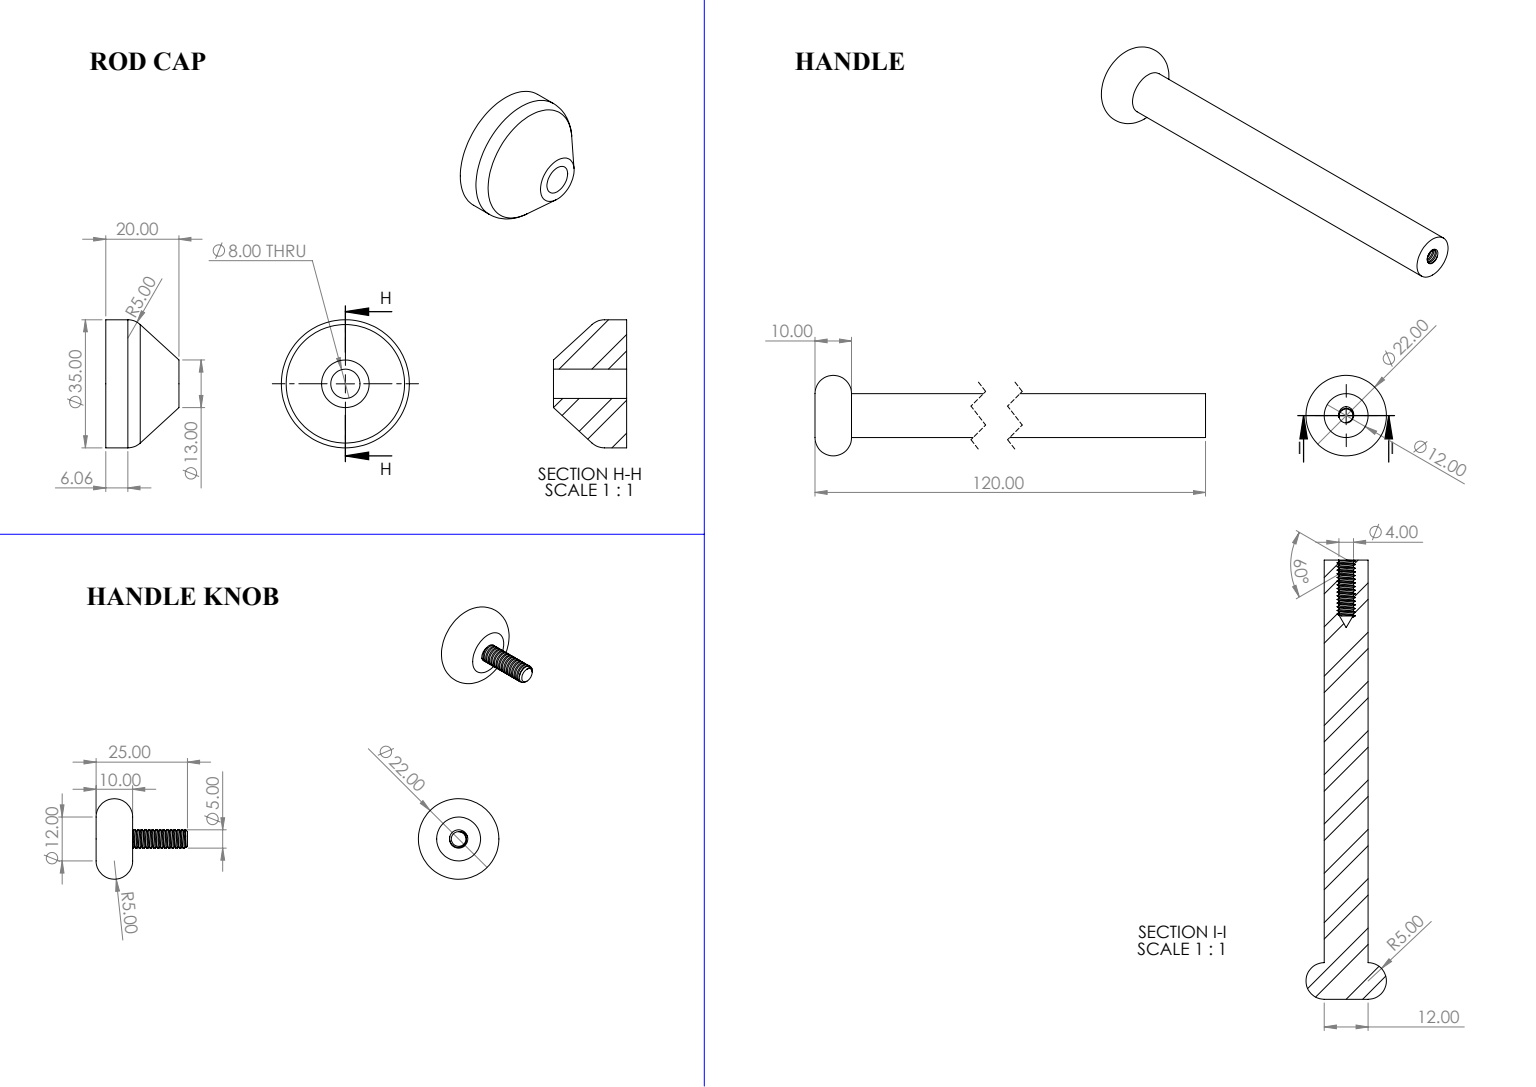
ISO-10303-21;
HEADER;
FILE_DESCRIPTION (('STEP AP214'),
    '1' );
FILE_NAME ('Handle knob.step',
    '2026-10-07T06:38:26',
    ( '' ),
    ( '' ),
    'SwSTEP 2.0',
    'SolidWorks 2021',
    '' );
FILE_SCHEMA (( 'AUTOMOTIVE_DESIGN' ));
ENDSEC;

DATA;
#8=CARTESIAN_POINT ( 'NONE',  ( 11.81249999999999822, -2.649519052838298805, 1.097466725451559322 ) ) ;
#12=CARTESIAN_POINT ( 'NONE',  ( 18.18750000000005684, 0.8284271247463557142, 1.999999999999971800 ) ) ;
#24=CARTESIAN_POINT ( 'NONE',  ( 15.64882486540532547, 2.500000000000084821, -1.035533905932929599 ) ) ;
#43=VECTOR ( 'NONE', #27184, 1000.000000000000000 ) ;
#80=SURFACE_SIDE_STYLE ('',( #6693 ) ) ;
#85=CARTESIAN_POINT ( 'NONE',  ( 19.25000000000009948, 1.110223024625156540E-13, 1.999999999999946265 ) ) ;
#100=CARTESIAN_POINT ( 'NONE',  ( 23.03867513459492855, 2.220446049250313081E-13, -2.500000000000057732 ) ) ;
#114=CARTESIAN_POINT ( 'NONE',  ( 9.937500000000083489, -1.097466725451379244, 2.649519052838238409 ) ) ;
#115=UNCERTAINTY_MEASURE_WITH_UNIT (LENGTH_MEASURE( 1.000000000000000082E-05 ), #12056, 'distance_accuracy_value', 'NONE');
#119=CARTESIAN_POINT ( 'NONE',  ( 23.66367513459491434, -1.767766952966209892, 1.767766952966376426 ) ) ;
#123=ORIENTED_EDGE ( 'NONE', *, *, #24115, .F. ) ;
#129=CARTESIAN_POINT ( 'NONE',  ( 21.62500000000011724, 1.110223024625156540E-13, 2.649519052838167354 ) ) ;
#153=CARTESIAN_POINT ( 'NONE',  ( 21.25000000000013145, -1.873492889144845464, -1.873492889145178530 ) ) ;
#161=CARTESIAN_POINT ( 'NONE',  ( 22.21132486540528106, -2.499999999999780176, -1.110223024625156540E-13 ) ) ;
#166=CARTESIAN_POINT ( 'NONE',  ( 20.85117513459493921, -2.499999999999844569, -1.035533905932809473 ) ) ;
#173=CARTESIAN_POINT ( 'NONE',  ( 19.75000000000009948, 1.665334536937734811E-13, -2.000000000000001776 ) ) ;
#178=CARTESIAN_POINT ( 'NONE',  ( 13.03867513459488947, 5.551115123125782702E-14, -2.500000000000002220 ) ) ;
#220=CARTESIAN_POINT ( 'NONE',  ( 16.37500000000008527, -1.414213562373090038, 1.414213562373034527 ) ) ;
#223=FACE_OUTER_BOUND ( 'NONE', #11618, .T. ) ;
#232=CARTESIAN_POINT ( 'NONE',  ( 22.87500000000000711, 1.414213562373312083, -1.414213562373090038 ) ) ;
#256=CARTESIAN_POINT ( 'NONE',  ( 13.83632486540523132, 1.767766952966376426, 1.767766952966376426 ) ) ;
#260=CARTESIAN_POINT ( 'NONE',  ( 23.37500000000000711, -1.414213562373090038, 1.414213562373034527 ) ) ;
#262=EDGE_CURVE ( 'NONE', #25850, #8065, #1532, .T. ) ;
#274=STYLED_ITEM ( 'NONE', ( #25687 ), #21644 ) ;
#276=CARTESIAN_POINT ( 'NONE',  ( 19.25000000000009948, 1.873492889145067508, -1.873492889144956486 ) ) ;
#295=CARTESIAN_POINT ( 'NONE',  ( 17.56250000000009592, 2.649519052838419153, -1.097466725451619718 ) ) ;
#305=VERTEX_POINT ( 'NONE', #20290 ) ;
#315=CARTESIAN_POINT ( 'NONE',  ( 10.25000000000000888, 1.873492889144956486, -1.873492889144900975 ) ) ;
#317=CARTESIAN_POINT ( 'NONE',  ( 19.31250000000010303, -0.8284271247459350507, 2.000000000000091926 ) ) ;
#335=PRESENTATION_STYLE_ASSIGNMENT (( #28879 ) ) ;
#377=CARTESIAN_POINT ( 'NONE',  ( 20.25000000000015632, 1.110223024625156540E-13, 1.999999999999946265 ) ) ;
#408=DIRECTION ( 'NONE',  ( -8.326672684688675286E-17, -2.081668171172168821E-17, 1.000000000000000000 ) ) ;
#416=CARTESIAN_POINT ( 'NONE',  ( 18.12500000000011369, 1.110223024625156540E-13, -2.649519052838278377 ) ) ;
#443=EDGE_LOOP ( 'NONE', ( #123, #12542, #25078, #1896 ) ) ;
#455=CARTESIAN_POINT ( 'NONE',  ( 10.93750000000009948, 2.000000000000091926, -0.8284271247462354770 ) ) ;
#456=ORIENTED_EDGE ( 'NONE', *, *, #9428, .T. ) ;
#458=CARTESIAN_POINT ( 'NONE',  ( 12.37500000000010836, 2.649519052838500421, 0.000000000000000000 ) ) ;
#462=CARTESIAN_POINT ( 'NONE',  ( 20.43750000000014566, -1.999999999999911626, 0.8284271247462354770 ) ) ;
#465=CARTESIAN_POINT ( 'NONE',  ( 22.97617513459487881, -1.035533905932689347, -2.500000000000024425 ) ) ;
#473=EDGE_CURVE ( 'NONE', #2749, #5395, #21945, .T. ) ;
#475=CARTESIAN_POINT ( 'NONE',  ( 15.71132486540535744, 2.500000000000113243, -1.110223024625156540E-13 ) ) ;
#482=CARTESIAN_POINT ( 'NONE',  ( 11.93750000000008527, 2.000000000000091926, -0.8284271247462354770 ) ) ;
#526=CARTESIAN_POINT ( 'NONE',  ( 22.00000000000010303, 2.000000000000168310, 0.000000000000000000 ) ) ;
#531=AXIS2_PLACEMENT_3D ( 'NONE', #29230, #26925, #12705 ) ;
#532=EDGE_CURVE ( 'NONE', #23217, #14931, #6701, .T. ) ;
#554=CARTESIAN_POINT ( 'NONE',  ( 23.50000000000010303, -1.999999999999779732, -5.551115123125782702E-14 ) ) ;
#566=VERTEX_POINT ( 'NONE', #11935 ) ;
#569=CARTESIAN_POINT ( 'NONE',  ( 16.87499999999997158, -2.649519052838222866, 0.000000000000000000 ) ) ;
#576=AXIS2_PLACEMENT_3D ( 'NONE', #8205, #17621, #15159 ) ;
#595=ORIENTED_EDGE ( 'NONE', *, *, #5857, .F. ) ;
#599=( BOUNDED_CURVE ( )  B_SPLINE_CURVE ( 2, ( #12471, #25953, #21667, #4903, #7659, #2902, #14759, #17068, #757 ),
 .UNSPECIFIED., .F., .T. ) 
 B_SPLINE_CURVE_WITH_KNOTS ( ( 3, 2, 2, 2, 3 ),
 ( 0.4531250000000000000, 0.4609375000000000000, 0.4687500000000000000, 0.4765625000000000000, 0.4843750000000000000 ),
 .UNSPECIFIED. ) 
 CURVE ( )  GEOMETRIC_REPRESENTATION_ITEM ( )  RATIONAL_B_SPLINE_CURVE ( ( 1.000000000000000000, 0.9238795325112867385, 1.000000000000000000, 0.9238795325112867385, 1.000000000000000000, 0.9238795325112867385, 1.000000000000000000, 0.9238795325112867385, 1.000000000000000000 ) ) 
 REPRESENTATION_ITEM ( '' )  );
#604=CARTESIAN_POINT ( 'NONE',  ( 22.58632486540529527, 1.767766952966487448, -1.767766952966431937 ) ) ;
#611=CARTESIAN_POINT ( 'NONE',  ( 11.12500000000010658, 1.414213562373201061, 1.414213562373034527 ) ) ;
#620=CARTESIAN_POINT ( 'NONE',  ( 20.75000000000012790, 1.665334536937734811E-13, -2.000000000000001776 ) ) ;
#623=CARTESIAN_POINT ( 'NONE',  ( 10.00000000000014744, 1.110223024625156540E-13, -5.551115123125782702E-14 ) ) ;
#625=CARTESIAN_POINT ( 'NONE',  ( -2.081668171172168020E-16, -5.204170427930420051E-17, 2.499999999999999112 ) ) ;
#626=CARTESIAN_POINT ( 'NONE',  ( 15.53867513459491967, 1.110223024625156540E-13, 2.499999999999835687 ) ) ;
#641=CARTESIAN_POINT ( 'NONE',  ( 12.06249999999996447, 2.000000000000091926, 0.8284271247461753029 ) ) ;
#644=CARTESIAN_POINT ( 'NONE',  ( 20.46132486540533435, 1.110223024625156540E-13, -2.500000000000057732 ) ) ;
#675=CARTESIAN_POINT ( 'NONE',  ( 17.31250000000004263, -0.8284271247461152399, 2.000000000000091926 ) ) ;
#687=CARTESIAN_POINT ( 'NONE',  ( 23.00000000000013145, 2.000000000000168310, 0.000000000000000000 ) ) ;
#699=( NAMED_UNIT ( * ) SI_UNIT ( $, .STERADIAN. ) SOLID_ANGLE_UNIT ( ) );
#710=CARTESIAN_POINT ( 'NONE',  ( 24.87500000000009237, 1.414213562373312083, -1.414213562373145550 ) ) ;
#725=CARTESIAN_POINT ( 'NONE',  ( 20.18750000000012079, 1.097466725451679892, -2.649519052838238409 ) ) ;
#736=ORIENTED_EDGE ( 'NONE', *, *, #27454, .T. ) ;
#751=CARTESIAN_POINT ( 'NONE',  ( 17.06250000000010303, -2.649519052838178457, 1.097466725451559322 ) ) ;
#757=CARTESIAN_POINT ( 'NONE',  ( 17.53867513459494987, 1.665334536937734811E-13, 2.499999999999946709 ) ) ;
#760=ORIENTED_EDGE ( 'NONE', *, *, #21946, .T. ) ;
#773=CARTESIAN_POINT ( 'NONE',  ( 17.00000000000015277, 2.000000000000112799, 0.000000000000000000 ) ) ;
#809=EDGE_CURVE ( 'NONE', #26790, #13355, #14385, .T. ) ;
#829=CARTESIAN_POINT ( 'NONE',  ( 17.06250000000001066, 2.000000000000151879, 0.8284271247461753029 ) ) ;
#833=CARTESIAN_POINT ( 'NONE',  ( 15.50000000000023626, 1.873492889145123019, 1.873492889144845464 ) ) ;
#835=EDGE_CURVE ( 'NONE', #29880, #28765, #16801, .T. ) ;
#861=CARTESIAN_POINT ( 'NONE',  ( 18.81250000000011013, -2.649519052838178457, 1.097466725451379244 ) ) ;
#881=DIRECTION ( 'NONE',  ( -1.000000000000000000, -1.665334536937731113E-16, 1.526556658859586792E-16 ) ) ;
#886=VERTEX_POINT ( 'NONE', #10157 ) ;
#887=CARTESIAN_POINT ( 'NONE',  ( 19.18750000000007461, -2.649519052838178457, -1.097466725451499370 ) ) ;
#920=CARTESIAN_POINT ( 'NONE',  ( 13.08632486540528461, -1.767766952966265404, 1.767766952966320915 ) ) ;
#930=CARTESIAN_POINT ( 'NONE',  ( 11.21132486540529705, -2.499999999999891198, -5.551115123125782702E-14 ) ) ;
#935=CARTESIAN_POINT ( 'NONE',  ( 25.25000000000015987, 1.873492889145067508, -1.873492889144956486 ) ) ;
#937=DIRECTION ( 'NONE',  ( -8.326672684688675286E-17, -2.081668171172168821E-17, 1.000000000000000000 ) ) ;
#971=CARTESIAN_POINT ( 'NONE',  ( 18.12500000000000355, 1.414213562373090038, 1.414213562373090038 ) ) ;
#981=DIRECTION ( 'NONE',  ( -8.326672684688675286E-17, -2.081668171172168821E-17, 1.000000000000000000 ) ) ;
#984=PLANE ( 'NONE',  #25487 ) ;
#996=CARTESIAN_POINT ( 'NONE',  ( 18.21132486540530238, -2.499999999999835687, -2.220446049250313081E-13 ) ) ;
#997=CARTESIAN_POINT ( 'NONE',  ( 10.77382486540524376, 2.499999999999964473, 1.035533905932689347 ) ) ;
#999=ORIENTED_EDGE ( 'NONE', *, *, #22038, .F. ) ;
#1028=DIRECTION ( 'NONE',  ( -1.000000000000000000, -1.665334536937731113E-16, 1.526556658859586792E-16 ) ) ;
#1035=( BOUNDED_CURVE ( )  B_SPLINE_CURVE ( 2, ( #20444, #22610, #6457, #17710, #18023, #8300, #10800, #6304, #22145 ),
 .UNSPECIFIED., .F., .T. ) 
 B_SPLINE_CURVE_WITH_KNOTS ( ( 3, 2, 2, 2, 3 ),
 ( 0.04687500000000000000, 0.05468750000000000000, 0.06250000000000000000, 0.07031250000000000000, 0.07812500000000000000 ),
 .UNSPECIFIED. ) 
 CURVE ( )  GEOMETRIC_REPRESENTATION_ITEM ( )  RATIONAL_B_SPLINE_CURVE ( ( 1.000000000000000000, 0.9238795325112867385, 1.000000000000000000, 0.9238795325112867385, 1.000000000000000000, 0.9238795325112867385, 1.000000000000000000, 0.9238795325112867385, 1.000000000000000000 ) ) 
 REPRESENTATION_ITEM ( '' )  );
#1038=CARTESIAN_POINT ( 'NONE',  ( 11.16367513459498539, 1.767766952966431937, -1.767766952966431937 ) ) ;
#1042=CARTESIAN_POINT ( 'NONE',  ( 13.50000000000006750, 1.873492889145123019, -1.873492889145011997 ) ) ;
#1084=CARTESIAN_POINT ( 'NONE',  ( 16.83632486540531659, 1.767766952966487448, 1.767766952966320915 ) ) ;
#1089=CARTESIAN_POINT ( 'NONE',  ( 10.43750000000004619, -1.999999999999851674, 0.8284271247461753029 ) ) ;
#1093=CARTESIAN_POINT ( 'NONE',  ( 20.96132486540536277, 5.551115123125782702E-14, 2.500000000000002220 ) ) ;
#1096=CARTESIAN_POINT ( 'NONE',  ( 10.06250000000005151, 2.000000000000212275, 0.8284271247461152399 ) ) ;
#1099=FACE_OUTER_BOUND ( 'NONE', #25635, .T. ) ;
#1113=CARTESIAN_POINT ( 'NONE',  ( 15.12500000000000000, 1.414213562373201061, 1.414213562373034527 ) ) ;
#1125=CARTESIAN_POINT ( 'NONE',  ( 15.31250000000006928, -0.8284271247461753029, 1.999999999999911626 ) ) ;
#1148=CARTESIAN_POINT ( 'NONE',  ( 10.89882486540524198, 1.035533905932749299, 2.499999999999904521 ) ) ;
#1155=ADVANCED_BREP_SHAPE_REPRESENTATION ( '', ( #4002, #18805 ), #12932 ) ;
#1156=( BOUNDED_CURVE ( )  B_SPLINE_CURVE ( 2, ( #15701, #3965, #25011, #22735, #10302, #12938, #19665, #29006, #22274 ),
 .UNSPECIFIED., .F., .F. ) 
 B_SPLINE_CURVE_WITH_KNOTS ( ( 3, 2, 2, 2, 3 ),
 ( 0.2656250000000000000, 0.2734375000000000000, 0.2812500000000000000, 0.2890625000000000000, 0.2968750000000000000 ),
 .UNSPECIFIED. ) 
 CURVE ( )  GEOMETRIC_REPRESENTATION_ITEM ( )  RATIONAL_B_SPLINE_CURVE ( ( 1.000000000000000000, 0.9238795325112867385, 1.000000000000000000, 0.9238795325112867385, 1.000000000000000000, 0.9238795325112867385, 1.000000000000000000, 0.9238795325112867385, 1.000000000000000000 ) ) 
 REPRESENTATION_ITEM ( '' )  );
#1171=CARTESIAN_POINT ( 'NONE',  ( 10.27382486540518869, -2.499999999999844569, -1.035533905932809473 ) ) ;
#1182=CARTESIAN_POINT ( 'NONE',  ( 14.68750000000004796, 2.649519052838478661, 1.097466725451439196 ) ) ;
#1194=VERTEX_POINT ( 'NONE', #13469 ) ;
#1202=CARTESIAN_POINT ( 'NONE',  ( 14.81250000000010658, 0.8284271247463557142, -2.000000000000031530 ) ) ;
#1221=CARTESIAN_POINT ( 'NONE',  ( 24.12500000000011724, -2.649519052838167354, 0.000000000000000000 ) ) ;
#1225=ADVANCED_FACE ( 'NONE', ( #2223 ), #14094, .T. ) ;
#1232=CARTESIAN_POINT ( 'NONE',  ( 19.53867513459495342, 5.551115123125782702E-14, 2.500000000000002220 ) ) ;
#1239=CARTESIAN_POINT ( 'NONE',  ( 24.62500000000000711, 1.110223024625156540E-13, 2.649519052838056332 ) ) ;
#1242=CARTESIAN_POINT ( 'NONE',  ( 2.081668171172167281E-16, 3.582034040661430693E-16, -2.499999999999999112 ) ) ;
#1267=CARTESIAN_POINT ( 'NONE',  ( 15.93749999999996980, 2.000000000000091926, -0.8284271247462955401 ) ) ;
#1275=B_SPLINE_CURVE_WITH_KNOTS ( 'NONE', 3,
 ( #25498, #22914, #30115, #6462, #15730, #4464, #25040, #13891, #15888, #15580, #24893, #11260, #11103, #29807, #23230, #3842, #22615, #20610 ),
 .UNSPECIFIED., .F., .F.,
 ( 4, 2, 2, 2, 2, 2, 2, 2, 4 ),
 ( 0.001391798398341157015, 0.001904360710870518173, 0.002416923023399879331, 0.002929485335929240489, 0.003442047648458601648, 0.003954609960987962372, 0.004467172273517323530, 0.004979734586046684688, 0.005492296898576045847 ),
 .UNSPECIFIED. ) ;
#1278=CARTESIAN_POINT ( 'NONE',  ( 18.18750000000005684, 0.8284271247463557142, 1.999999999999971800 ) ) ;
#1298=( BOUNDED_CURVE ( )  B_SPLINE_CURVE ( 2, ( #8723, #27280, #10584, #3789, #10750, #8562, #6254, #15672, #29438 ),
 .UNSPECIFIED., .F., .T. ) 
 B_SPLINE_CURVE_WITH_KNOTS ( ( 3, 2, 2, 2, 3 ),
 ( 0.2031250000000000000, 0.2109375000000000000, 0.2187500000000000000, 0.2265625000000000000, 0.2343750000000000000 ),
 .UNSPECIFIED. ) 
 CURVE ( )  GEOMETRIC_REPRESENTATION_ITEM ( )  RATIONAL_B_SPLINE_CURVE ( ( 1.000000000000000000, 0.9238795325112867385, 1.000000000000000000, 0.9238795325112867385, 1.000000000000000000, 0.9238795325112867385, 1.000000000000000000, 0.9238795325112867385, 1.000000000000000000 ) ) 
 REPRESENTATION_ITEM ( '' )  );
#1310=CARTESIAN_POINT ( 'NONE',  ( 0.000000000000000000, 0.000000000000000000, 0.000000000000000000 ) ) ;
#1314=UNCERTAINTY_MEASURE_WITH_UNIT (LENGTH_MEASURE( 1.000000000000000082E-05 ), #17406, 'distance_accuracy_value', 'NONE');
#1327=CARTESIAN_POINT ( 'NONE',  ( 22.66367513459499605, -1.767766952966265404, 1.767766952966376426 ) ) ;
#1338=CARTESIAN_POINT ( 'NONE',  ( 23.89882486540529882, 1.035533905932809473, 2.499999999999844569 ) ) ;
#1344=CARTESIAN_POINT ( 'NONE',  ( 14.50000000000012434, 1.873492889145067508, -1.873492889144956486 ) ) ;
#1370=CARTESIAN_POINT ( 'NONE',  ( 16.68750000000013856, -0.8284271247461753029, -2.000000000000151879 ) ) ;
#1385=CARTESIAN_POINT ( 'NONE',  ( 17.72617513459489658, -2.499999999999964473, 1.035533905932749299 ) ) ;
#1393=CARTESIAN_POINT ( 'NONE',  ( 19.72617513459489658, -2.499999999999964473, 1.035533905932809473 ) ) ;
#1417=CARTESIAN_POINT ( 'NONE',  ( 10.35117513459487704, 2.500000000000084821, 1.035533905932689347 ) ) ;
#1427=CARTESIAN_POINT ( 'NONE',  ( 14.68750000000004796, -0.8284271247460552878, -1.999999999999971800 ) ) ;
#1428=ORIENTED_EDGE ( 'NONE', *, *, #835, .F. ) ;
#1439=CARTESIAN_POINT ( 'NONE',  ( 15.81250000000000000, 0.8284271247462354770, -2.000000000000151879 ) ) ;
#1442=CARTESIAN_POINT ( 'NONE',  ( 14.68749999999998579, -1.097466725451499370, 2.649519052838298805 ) ) ;
#1469=ORIENTED_EDGE ( 'NONE', *, *, #28809, .T. ) ;
#1494=CARTESIAN_POINT ( 'NONE',  ( 15.81250000000009237, 1.097466725451619718, 2.649519052838419153 ) ) ;
#1507=AXIS2_PLACEMENT_3D ( 'NONE', #7070, #30110, #16484 ) ;
#1520=CARTESIAN_POINT ( 'NONE',  ( 13.25000000000017764, 5.551115123125782702E-14, 1.999999999999890754 ) ) ;
#1524=VECTOR ( 'NONE', #23636, 1000.000000000000000 ) ;
#1532=LINE ( 'NONE', #1995, #6368 ) ;
#1536=ORIENTED_EDGE ( 'NONE', *, *, #23552, .F. ) ;
#1537=CARTESIAN_POINT ( 'NONE',  ( 24.25000000000010658, -1.873492889144789952, -1.873492889145123019 ) ) ;
#1561=CARTESIAN_POINT ( 'NONE',  ( 24.43750000000014921, -1.999999999999851674, 0.8284271247462354770 ) ) ;
#1573=CARTESIAN_POINT ( 'NONE',  ( 14.22617513459491256, 2.500000000000144773, -1.035533905932689347 ) ) ;
#1574=VERTEX_POINT ( 'NONE', #20789 ) ;
#1578=( BOUNDED_CURVE ( )  B_SPLINE_CURVE ( 2, ( #24390, #7794, #1038, #19787, #25134, #13365, #5946, #20258, #27140 ),
 .UNSPECIFIED., .F., .T. ) 
 B_SPLINE_CURVE_WITH_KNOTS ( ( 3, 2, 2, 2, 3 ),
 ( 0.07812500000000000000, 0.08593750000000000000, 0.09375000000000000000, 0.1015625000000000000, 0.1093750000000000000 ),
 .UNSPECIFIED. ) 
 CURVE ( )  GEOMETRIC_REPRESENTATION_ITEM ( )  RATIONAL_B_SPLINE_CURVE ( ( 1.000000000000000000, 0.9238795325112867385, 1.000000000000000000, 0.9238795325112867385, 1.000000000000000000, 0.9238795325112867385, 1.000000000000000000, 0.9238795325112867385, 1.000000000000000000 ) ) 
 REPRESENTATION_ITEM ( '' )  );
#1583=AXIS2_PLACEMENT_3D ( 'NONE', #28607, #19132, #14405 ) ;
#1594=CARTESIAN_POINT ( 'NONE',  ( 13.75000000000006750, 2.220446049250313081E-13, -2.000000000000001776 ) ) ;
#1597=CARTESIAN_POINT ( 'NONE',  ( 14.43750000000004974, 2.649519052838419153, 1.097466725451439196 ) ) ;
#1606=CARTESIAN_POINT ( 'NONE',  ( 17.89882486540517093, 1.035533905932749299, 2.499999999999964473 ) ) ;
#1612=TOROIDAL_SURFACE ( 'NONE', #14425, 6.000000000000000888, 5.000000000000000888 ) ;
#1617=CARTESIAN_POINT ( 'NONE',  ( 20.81250000000014211, 0.8284271247461753029, -2.000000000000091926 ) ) ;
#1626=ORIENTED_EDGE ( 'NONE', *, *, #5088, .F. ) ;
#1628=CARTESIAN_POINT ( 'NONE',  ( 16.68750000000013856, -1.097466725451439196, 2.649519052838178457 ) ) ;
#1636=ORIENTED_EDGE ( 'NONE', *, *, #13213, .F. ) ;
#1654=CARTESIAN_POINT ( 'NONE',  ( 14.06250000000011546, -2.649519052838238409, 1.097466725451559322 ) ) ;
#1691=EDGE_CURVE ( 'NONE', #24822, #4865, #27940, .T. ) ;
#1702=CARTESIAN_POINT ( 'NONE',  ( 15.02382486540530238, -1.035533905932568999, 2.499999999999784173 ) ) ;
#1714=CARTESIAN_POINT ( 'NONE',  ( 22.31250000000002842, -0.8284271247460552878, 2.000000000000031530 ) ) ;
#1721=CARTESIAN_POINT ( 'NONE',  ( 12.03867513459491789, 1.665334536937734811E-13, -2.500000000000057732 ) ) ;
#1727=CYLINDRICAL_SURFACE ( 'NONE', #6676, 2.499999999999999112 ) ;
#1742=CARTESIAN_POINT ( 'NONE',  ( 11.93750000000008527, 2.000000000000091926, -0.8284271247462354770 ) ) ;
#1744=EDGE_CURVE ( 'NONE', #13355, #26790, #5902, .T. ) ;
#1746=CARTESIAN_POINT ( 'NONE',  ( 18.16367513459488237, 1.767766952966487448, -1.767766952966487448 ) ) ;
#1752=CARTESIAN_POINT ( 'NONE',  ( 0.000000000000000000, 0.000000000000000000, 0.000000000000000000 ) ) ;
#1767=CARTESIAN_POINT ( 'NONE',  ( 20.12500000000011369, 1.414213562373201061, 1.414213562373034527 ) ) ;
#1773=CARTESIAN_POINT ( 'NONE',  ( 14.77382486540530770, 2.500000000000144773, 1.035533905932689347 ) ) ;
#1778=EDGE_LOOP ( 'NONE', ( #21927, #2761, #24888, #28248 ) ) ;
#1793=CARTESIAN_POINT ( 'NONE',  ( 10.39882486540515849, -1.035533905932629173, -2.500000000000024425 ) ) ;
#1802=CARTESIAN_POINT ( 'NONE',  ( 11.62500000000010658, 2.649519052838444910, -1.110223024625156540E-13 ) ) ;
#1806=VERTEX_POINT ( 'NONE', #14612 ) ;
#1817=EDGE_CURVE ( 'NONE', #9159, #21560, #599, .T. ) ;
#1819=CARTESIAN_POINT ( 'NONE',  ( 10.37500000000005151, -1.414213562373034527, 1.414213562372756972 ) ) ;
#1828=CARTESIAN_POINT ( 'NONE',  ( 11.62499999999999645, -1.414213562373090038, -1.414213562373090038 ) ) ;
#1846=CARTESIAN_POINT ( 'NONE',  ( 21.12500000000011724, -2.649519052838222866, 0.000000000000000000 ) ) ;
#1866=CARTESIAN_POINT ( 'NONE',  ( 23.56250000000009948, -1.999999999999851674, -0.8284271247462354770 ) ) ;
#1879=DIRECTION ( 'NONE',  ( -1.000000000000000000, -1.665334536937731113E-16, 1.526556658859586792E-16 ) ) ;
#1893=SHAPE_REPRESENTATION ( 'Handle knob', ( #18805 ), #12932 ) ;
#1896=ORIENTED_EDGE ( 'NONE', *, *, #30228, .T. ) ;
#1897=CARTESIAN_POINT ( 'NONE',  ( 13.37500000000019185, -1.414213562372979016, 1.414213562372979016 ) ) ;
#1902=CARTESIAN_POINT ( 'NONE',  ( 10.31249999999998934, -0.8284271247461753029, 1.999999999999911626 ) ) ;
#1924=CARTESIAN_POINT ( 'NONE',  ( 19.68750000000015632, -0.8284271247461152399, -1.999999999999971800 ) ) ;
#1952=CARTESIAN_POINT ( 'NONE',  ( 23.41367513459491434, 1.767766952966487448, 1.767766952966098870 ) ) ;
#1963=CARTESIAN_POINT ( 'NONE',  ( 10.43750000000010658, 1.097466725451619718, -2.649519052838358757 ) ) ;
#1966=CARTESIAN_POINT ( 'NONE',  ( 16.53867513459489302, 5.551115123125782702E-14, 2.500000000000002220 ) ) ;
#1977=CARTESIAN_POINT ( 'NONE',  ( 23.81250000000003553, -2.649519052838298805, 1.097466725451559322 ) ) ;
#1979=EDGE_LOOP ( 'NONE', ( #12993, #26078, #15721, #25258 ) ) ;
#1995=CARTESIAN_POINT ( 'NONE',  ( -2.081668171172168020E-16, -5.204170427930420051E-17, 2.499999999999999112 ) ) ;
#2003=CARTESIAN_POINT ( 'NONE',  ( 20.68750000000014211, 2.649519052838478661, 1.097466725451559322 ) ) ;
#2015=CYLINDRICAL_SURFACE ( 'NONE', #15261, 2.499999999999999112 ) ;
#2026=CARTESIAN_POINT ( 'NONE',  ( 22.06250000000015632, 2.000000000000212275, 0.8284271247461753029 ) ) ;
#2035=CARTESIAN_POINT ( 'NONE',  ( 12.35117513459494099, 2.500000000000084821, 1.035533905932749299 ) ) ;
#2044=ORIENTED_EDGE ( 'NONE', *, *, #19178, .T. ) ;
#2057=CARTESIAN_POINT ( 'NONE',  ( 12.50000000000012257, -1.999999999999835243, 0.000000000000000000 ) ) ;
#2058=DIRECTION ( 'NONE',  ( -1.000000000000000000, -1.665334536937731113E-16, 1.526556658859586792E-16 ) ) ;
#2065=CARTESIAN_POINT ( 'NONE',  ( 13.62500000000016520, -1.414213562372923505, -1.414213562373145550 ) ) ;
#2109=VECTOR ( 'NONE', #6636, 1000.000000000000000 ) ;
#2122=CARTESIAN_POINT ( 'NONE',  ( 10.87500000000010658, 5.551115123125782702E-14, 2.649519052838056332 ) ) ;
#2132=( BOUNDED_CURVE ( )  B_SPLINE_CURVE ( 2, ( #30291, #12051, #23698, #14064, #475, #24, #9252, #12205, #19097 ),
 .UNSPECIFIED., .F., .T. ) 
 B_SPLINE_CURVE_WITH_KNOTS ( ( 3, 2, 2, 2, 3 ),
 ( 0.5468750000000000000, 0.5546875000000000000, 0.5625000000000000000, 0.5703125000000000000, 0.5781250000000000000 ),
 .UNSPECIFIED. ) 
 CURVE ( )  GEOMETRIC_REPRESENTATION_ITEM ( )  RATIONAL_B_SPLINE_CURVE ( ( 1.000000000000000000, 0.9238795325112867385, 1.000000000000000000, 0.9238795325112867385, 1.000000000000000000, 0.9238795325112867385, 1.000000000000000000, 0.9238795325112867385, 1.000000000000000000 ) ) 
 REPRESENTATION_ITEM ( '' )  );
#2138=CARTESIAN_POINT ( 'NONE',  ( 23.00000000000007461, -1.873492889144900975, -1.873492889144956486 ) ) ;
#2146=EDGE_CURVE ( 'NONE', #21560, #26328, #3356, .T. ) ;
#2148=CARTESIAN_POINT ( 'NONE',  ( 10.93750000000009948, 2.000000000000091926, -0.8284271247462354770 ) ) ;
#2163=FACE_OUTER_BOUND ( 'NONE', #5498, .T. ) ;
#2178=CARTESIAN_POINT ( 'NONE',  ( 24.50000000000010658, 5.551115123125782702E-14, -5.551115123125782702E-14 ) ) ;
#2181=CARTESIAN_POINT ( 'NONE',  ( 22.81250000000002132, 0.8284271247461753029, -2.000000000000091926 ) ) ;
#2187=FACE_OUTER_BOUND ( 'NONE', #8745, .T. ) ;
#2209=CARTESIAN_POINT ( 'NONE',  ( 13.96132486540527218, 1.110223024625156540E-13, 2.499999999999946709 ) ) ;
#2212=CARTESIAN_POINT ( 'NONE',  ( 14.81250000000010481, 0.8284271247463557142, -2.000000000000031530 ) ) ;
#2217=CARTESIAN_POINT ( 'NONE',  ( 18.89882486540528106, 1.035533905932809473, 2.499999999999844569 ) ) ;
#2223=FACE_OUTER_BOUND ( 'NONE', #28038, .T. ) ;
#2225=TOROIDAL_SURFACE ( 'NONE', #19378, 6.000000000000000888, 5.000000000000000888 ) ;
#2242=CARTESIAN_POINT ( 'NONE',  ( 19.93750000000015277, 2.000000000000091926, -0.8284271247462354770 ) ) ;
#2243=VECTOR ( 'NONE', #6829, 1000.000000000000000 ) ;
#2250=CARTESIAN_POINT ( 'NONE',  ( 11.83632486540522954, 1.767766952966431937, 1.767766952966098870 ) ) ;
#2256=ADVANCED_FACE ( 'NONE', ( #30410 ), #27296, .T. ) ;
#2274=ORIENTED_EDGE ( 'NONE', *, *, #28192, .T. ) ;
#2278=( BOUNDED_CURVE ( )  B_SPLINE_CURVE ( 2, ( #18950, #12200, #9711, #16942, #21541, #21832, #16805, #28710, #626 ),
 .UNSPECIFIED., .F., .F. ) 
 B_SPLINE_CURVE_WITH_KNOTS ( ( 3, 2, 2, 2, 3 ),
 ( 0.3281250000000000000, 0.3359375000000000000, 0.3437500000000000000, 0.3515625000000000000, 0.3593750000000000000 ),
 .UNSPECIFIED. ) 
 CURVE ( )  GEOMETRIC_REPRESENTATION_ITEM ( )  RATIONAL_B_SPLINE_CURVE ( ( 1.000000000000000000, 0.9238795325112867385, 1.000000000000000000, 0.9238795325112867385, 1.000000000000000000, 0.9238795325112867385, 1.000000000000000000, 0.9238795325112867385, 1.000000000000000000 ) ) 
 REPRESENTATION_ITEM ( '' )  );
#2289=ORIENTED_EDGE ( 'NONE', *, *, #28821, .T. ) ;
#2291=CARTESIAN_POINT ( 'NONE',  ( 20.62500000000008882, 5.551115123125782702E-14, 2.649519052838056332 ) ) ;
#2300=CARTESIAN_POINT ( 'NONE',  ( 10.50000000000003730, -1.999999999999835243, 0.000000000000000000 ) ) ;
#2312=ORIENTED_EDGE ( 'NONE', *, *, #7278, .F. ) ;
#2314=CARTESIAN_POINT ( 'NONE',  ( 21.68750000000007105, 2.649519052838419153, 1.097466725451559322 ) ) ;
#2329=CARTESIAN_POINT ( 'NONE',  ( 20.91367513459485394, -1.767766952966154381, -1.767766952966487448 ) ) ;
#2336=CARTESIAN_POINT ( 'NONE',  ( 18.87500000000008527, 1.414213562373256572, -1.414213562373090038 ) ) ;
#2342=CARTESIAN_POINT ( 'NONE',  ( 12.85117513459490191, -2.499999999999844569, -1.035533905932809473 ) ) ;
#2344=CARTESIAN_POINT ( 'NONE',  ( 24.65159914405371921, -2.238694682432001759, 0.7252922178121359309 ) ) ;
#2352=FACE_OUTER_BOUND ( 'NONE', #19071, .T. ) ;
#2398=CARTESIAN_POINT ( 'NONE',  ( 22.37500000000011724, -1.414213562372979016, 1.414213562372979016 ) ) ;
#2411=CARTESIAN_POINT ( 'NONE',  ( 24.99999999999999289, 1.110223024625156540E-13, -2.220446049250313081E-13 ) ) ;
#2415=CARTESIAN_POINT ( 'NONE',  ( 21.39882486540530238, -1.035533905932749299, -2.499999999999964473 ) ) ;
#2418=CARTESIAN_POINT ( 'NONE',  ( 13.58632486540531303, 1.767766952966487448, -1.767766952966320915 ) ) ;
#2422=CARTESIAN_POINT ( 'NONE',  ( 10.06250000000008349, -2.649519052838178457, 1.097466725451499370 ) ) ;
#2426=CARTESIAN_POINT ( 'NONE',  ( 10.00000000000009059, 2.022462396512465510, -0.1718975768220544764 ) ) ;
#2430=CARTESIAN_POINT ( 'NONE',  ( 9.937500000000083489, 2.000000000000151879, -0.8284271247463557142 ) ) ;
#2440=CARTESIAN_POINT ( 'NONE',  ( 23.68750000000013500, -1.097466725451379244, 2.649519052838358757 ) ) ;
#2459=CARTESIAN_POINT ( 'NONE',  ( 21.93750000000006395, -1.097466725451379244, 2.649519052838178457 ) ) ;
#2475=CARTESIAN_POINT ( 'NONE',  ( 10.06250000000005151, -1.097466725451499370, -2.649519052838419153 ) ) ;
#2476=CARTESIAN_POINT ( 'NONE',  ( 19.93750000000015277, 2.000000000000091926, -0.8284271247462354770 ) ) ;
#2484=CARTESIAN_POINT ( 'NONE',  ( 24.58754953339359162, -1.405346041411892788, 1.966652551842076990 ) ) ;
#2528=CARTESIAN_POINT ( 'NONE',  ( 16.62500000000013856, -1.414213562372867994, -1.414213562373145550 ) ) ;
#2542=CARTESIAN_POINT ( 'NONE',  ( 20.75000000000012790, 1.665334536937734811E-13, -2.000000000000001776 ) ) ;
#2555=CARTESIAN_POINT ( 'NONE',  ( 21.02382486540522066, -1.035533905932749299, 2.499999999999964473 ) ) ;
#2563=CARTESIAN_POINT ( 'NONE',  ( 23.87500000000009237, 1.414213562373256572, -1.414213562373145550 ) ) ;
#2570=ORIENTED_EDGE ( 'NONE', *, *, #8367, .T. ) ;
#2578=CARTESIAN_POINT ( 'NONE',  ( 21.43750000000003908, 2.649519052838419153, 1.097466725451499370 ) ) ;
#2601=CARTESIAN_POINT ( 'NONE',  ( 19.31250000000007105, -1.097466725451379244, -2.649519052838538613 ) ) ;
#2613=ORIENTED_EDGE ( 'NONE', *, *, #2686, .T. ) ;
#2620=CARTESIAN_POINT ( 'NONE',  ( 10.56250000000013678, 1.097466725451679892, 2.649519052838419153 ) ) ;
#2622=CARTESIAN_POINT ( 'NONE',  ( 18.43749999999999289, -1.999999999999971800, 0.8284271247462354770 ) ) ;
#2631=CYLINDRICAL_SURFACE ( 'NONE', #9262, 2.499999999999999112 ) ;
#2633=EDGE_LOOP ( 'NONE', ( #12030, #17756, #23523, #12329 ) ) ;
#2641=CARTESIAN_POINT ( 'NONE',  ( 12.25000000000006573, 5.551115123125782702E-14, 1.999999999999946265 ) ) ;
#2654=PRODUCT_DEFINITION_CONTEXT ( 'detailed design', #14794, 'design' ) ;
#2681=CARTESIAN_POINT ( 'NONE',  ( 21.43750000000007105, -1.999999999999911626, 0.8284271247461753029 ) ) ;
#2683=ORIENTED_EDGE ( 'NONE', *, *, #3065, .T. ) ;
#2686=EDGE_CURVE ( 'NONE', #29417, #10444, #19362, .T. ) ;
#2705=DIRECTION ( 'NONE',  ( 0.000000000000000000, -2.081668171172248016E-17, 1.000000000000000000 ) ) ;
#2716=COLOUR_RGB ( '', 0.31764706, 0.68627451, 0.89019608) ;
#2718=CARTESIAN_POINT ( 'NONE',  ( 17.06250000000004263, -1.097466725451439196, -2.649519052838358757 ) ) ;
#2741=CARTESIAN_POINT ( 'NONE',  ( 18.43749999999990408, 1.097466725451619718, -2.649519052838358757 ) ) ;
#2745=CARTESIAN_POINT ( 'NONE',  ( 18.39882486540522422, -1.035533905932689347, -2.500000000000084821 ) ) ;
#2749=VERTEX_POINT ( 'NONE', #21554 ) ;
#2752=ADVANCED_FACE ( 'NONE', ( #10177 ), #2225, .T. ) ;
#2753=CARTESIAN_POINT ( 'NONE',  ( 22.83632486540521001, 1.767766952966376426, 1.767766952966376426 ) ) ;
#2755=CARTESIAN_POINT ( 'NONE',  ( 22.53867513459501026, 1.110223024625156540E-13, 2.499999999999835687 ) ) ;
#2756=EDGE_CURVE ( 'NONE', #566, #20580, #1035, .T. ) ;
#2761=ORIENTED_EDGE ( 'NONE', *, *, #5141, .T. ) ;
#2763=CARTESIAN_POINT ( 'NONE',  ( 12.18750000000008349, 1.097466725451679892, -2.649519052838238409 ) ) ;
#2764=CARTESIAN_POINT ( 'NONE',  ( 19.14882486540521356, -2.499999999999964473, 1.035533905932749299 ) ) ;
#2766=CARTESIAN_POINT ( 'NONE',  ( 19.06250000000013500, 2.000000000000091926, 0.8284271247461753029 ) ) ;
#2771=CARTESIAN_POINT ( 'NONE',  ( 22.60117513459491434, -1.035533905932629173, 2.499999999999784173 ) ) ;
#2782=( NAMED_UNIT ( * ) SI_UNIT ( $, .STERADIAN. ) SOLID_ANGLE_UNIT ( ) );
#2786=( NAMED_UNIT ( * ) SI_UNIT ( $, .STERADIAN. ) SOLID_ANGLE_UNIT ( ) );
#2787=CARTESIAN_POINT ( 'NONE',  ( 12.12500000000005329, 1.414213562373201061, 1.414213562373034527 ) ) ;
#2831=CARTESIAN_POINT ( 'NONE',  ( 11.53867513459497296, 5.551115123125782702E-14, 2.500000000000002220 ) ) ;
#2834=CARTESIAN_POINT ( 'NONE',  ( 22.43750000000002842, -1.999999999999851674, 0.8284271247462354770 ) ) ;
#2857=CARTESIAN_POINT ( 'NONE',  ( 24.37500000000014566, -1.414213562373034527, 1.414213562373034527 ) ) ;
#2870=CARTESIAN_POINT ( 'NONE',  ( 20.37500000000017053, 2.649519052838555933, 0.000000000000000000 ) ) ;
#2896=CARTESIAN_POINT ( 'NONE',  ( 16.62500000000008527, 2.649519052838444910, -1.110223024625156540E-13 ) ) ;
#2902=CARTESIAN_POINT ( 'NONE',  ( 17.35117513459481131, 2.500000000000084821, 1.035533905932689347 ) ) ;
#2911=CARTESIAN_POINT ( 'NONE',  ( 24.14882486540529527, -2.499999999999964473, 1.035533905932749299 ) ) ;
#2912=CARTESIAN_POINT ( 'NONE',  ( 10.87500000000005151, -2.649519052838111843, -5.551115123125782702E-14 ) ) ;
#2915=CARTESIAN_POINT ( 'NONE',  ( 19.68750000000015632, -0.8284271247461152399, -1.999999999999971800 ) ) ;
#2936=DIRECTION ( 'NONE',  ( 1.000000000000000000, 1.665334536937731113E-16, -1.526556658859586792E-16 ) ) ;
#2939=CARTESIAN_POINT ( 'NONE',  ( 20.89882486540530948, 1.035533905932809473, 2.499999999999844569 ) ) ;
#2956=EDGE_CURVE ( 'NONE', #28521, #23217, #28112, .T. ) ;
#2962=CARTESIAN_POINT ( 'NONE',  ( 10.03867513459497118, 1.110223024625156540E-13, -2.500000000000113243 ) ) ;
#2968=CARTESIAN_POINT ( 'NONE',  ( 17.37500000000011369, -1.414213562372979016, 1.414213562373034527 ) ) ;
#2978=CARTESIAN_POINT ( 'NONE',  ( 21.68750000000000711, -0.8284271247461753029, -2.000000000000031530 ) ) ;
#3002=CARTESIAN_POINT ( 'NONE',  ( 9.375000000000078160, 1.110223024625156540E-13, -2.649519052838444910 ) ) ;
#3007=( BOUNDED_SURFACE ( )  B_SPLINE_SURFACE ( 1, 2, ( 
 ( #19844, #3543, #13585, #6628, #30279, #20621, #22770, #29968, #6475, #1561, #8631, #8794, #27352, #22923, #22625, #20315, #18181, #11433, #25197, #6315, #4322, #29662, #18336, #1866, #6780, #6928, #23239, #11268, #23084, #25049, #20928, #15740, #18484, #16198, #29817, #2181, #27952, #11582, #27803, #20457, #13740, #3851, #8946, #1714, #15899, #4009, #10966, #2026, #20778, #13425, #9238, #27498, #18036, #25509, #9088, #11111, #4473, #18632, #4160, #27652, #16050, #30125, #25350, #13899, #16351, #13281, #26265, #23537, #620, #5216, #10005, #19380, #7526, #462, #14630, #18946, #16937, #11895, #4775, #23830, #28409, #2476, #25669, #23975, #173, #2915, #16649, #28704, #5064, #14493, #7675, #317, #4620, #9553, #14050, #2766, #23388, #21535, #2336, #28262, #11735, #19230, #25972, #9853, #21080, #2622, #4916, #14347, #28110, #12, #28558, #9397, #23685, #18789, #12043, #7084, #16498, #21381, #19089, #7390, #16798, #26118, #28861, #14772, #3511, #3204, #10304, #10154, #773, #27013, #5510, #22433, #5978, #1370, #10780, #8273, #22276, #15396, #19668, #24720, #21973, #26562, #15227, #19811, #24256, #17086, #3661, #29008, #20128, #7973, #29472, #26851, #5810, #26413, #22125, #5364, #17382, #24117, #24559, #3064, #12940, #12489, #26697, #1202, #5661, #24412, #19963, #21827, #14917, #10457, #15068, #17535, #3353, #19528, #7820, #12781, #17234, #10611, #29156, #8118, #30088, #8442, #8595, #18000, #11232, #20281, #27767, #4284, #1520, #11393, #6137, #9056, #6745, #6429, #20581, #4434, #25160, #27316, #4125, #11077, #15551, #13247, #13394, #29629, #13546, #27166, #24869, #22737, #16011, #8757, #15704, #18298, #25013, #22887, #1828, #20738, #11548, #16163, #29929, #27612, #3968, #25471, #20421, #13860, #23201, #2148, #20889, #17848, #4587, #27918, #18596, #14013, #2300, #10492, #1819, #4116, #15105, #3234, #7707, #1096, #17114, #29041, #29188, #26440, #3540, #12814, #10646, #12970, #6009 ),
 ( #12661, #22156, #935, #10184, #10337, #8007, #17414, #5693, #8149, #26884, #15263, #22307, #1239, #19997, #8310, #17720, #15427, #22877, #23496, #23645, #9513, #30233, #9354, #11385, #7194, #1977, #4731, #2440, #16153, #18900, #14305, #28221, #14159, #6734, #30386, #29921, #27909, #18439, #2138, #23034, #27601, #18746, #28067, #20728, #16605, #25461, #6580, #11850, #25783, #13696, #21188, #25926, #30079, #9047, #16003, #7043, #4425, #13853, #27756, #4274, #129, #23193, #4874, #2578, #8899, #25303, #11539, #20880, #9196, #18588, #6886, #25632, #4580, #16456, #23351, #14006, #2291, #11696, #21040, #3162, #2870, #24365, #21782, #725, #19621, #17036, #12001, #16894, #24213, #10110, #28964, #19479, #21333, #26213, #17189, #5169, #19336, #14870, #276, #28811, #7771, #7927, #26368, #9659, #14581, #861, #26512, #17337, #5463, #19049, #23933, #10261, #12291, #28655, #26653, #28365, #416, #5317, #9957, #12435, #7626, #5613, #7344, #7482, #16750, #26076, #5017, #14726, #14448, #23783, #12145, #21490, #24069, #2718, #9805, #28513, #569, #3019, #29110, #1628, #8707, #13047, #6085, #5765, #17797, #10560, #29586, #8546, #23608, #21296, #19148, #9619, #21599, #11970, #7310, #12404, #17152, #21896, #833, #10230, #24324, #22347, #15308, #29553, #11000, #27234, #17606, #27084, #29078, #24934, #8042, #1442, #6205, #12852, #15624, #1597, #13316, #22657, #24473, #17760, #17305, #24631, #5732, #19881, #26766, #5579, #6050, #3737, #22195, #20345, #10527, #14984, #26622, #13171, #29227, #3277, #3580, #13008, #20040, #8352, #7387, #7082, #14200, #14047, #4618, #21532, #9395, #16933, #458, #26262, #5213, #2763, #26115, #9849, #23535, #12191, #16496, #8, #19086, #23682, #28108, #20925, #19227, #25823, #28555, #11893, #23974, #12040, #21078, #23386, #14626, #7523, #2912, #30276, #9236, #18629, #27949, #2620, #4772, #9704, #6926, #5060, #315, #16349, #9551, #2475, #14345, #18944, #25668 ) ),
 .UNSPECIFIED., .F., .F., .F. ) 
 B_SPLINE_SURFACE_WITH_KNOTS ( ( 2, 2 ),
 ( 3, 2, 2, 2, 2, 2, 2, 2, 2, 2, 2, 2, 2, 2, 2, 2, 2, 2, 2, 2, 2, 2, 2, 2, 2, 2, 2, 2, 2, 2, 2, 2, 2, 2, 2, 2, 2, 2, 2, 2, 2, 2, 2, 2, 2, 2, 2, 2, 2, 2, 2, 2, 2, 2, 2, 2, 2, 2, 2, 2, 2, 2, 2, 2, 2, 2, 2, 2, 2, 2, 2, 2, 2, 2, 2, 2, 2, 2, 2, 2, 2, 2, 2, 2, 2, 2, 2, 2, 2, 2, 2, 2, 2, 2, 2, 2, 2, 2, 2, 2, 2, 2, 2, 2, 2, 2, 2, 2, 2, 2, 2, 2, 2, 2, 2, 2, 2, 2, 2, 2, 2, 2, 2, 2, 3 ),
 ( 0.000000000000000000, 1.000000000000000000 ),
 ( 0.000000000000000000, 0.007812500000000000000, 0.01562500000000000000, 0.02343750000000000000, 0.03125000000000000000, 0.03906250000000000000, 0.04687500000000000000, 0.05468750000000000000, 0.06250000000000000000, 0.07031250000000000000, 0.07812500000000000000, 0.08593750000000000000, 0.09375000000000000000, 0.1015625000000000000, 0.1093750000000000000, 0.1171875000000000000, 0.1250000000000000000, 0.1328125000000000000, 0.1406250000000000000, 0.1484375000000000000, 0.1562500000000000000, 0.1640625000000000000, 0.1718750000000000000, 0.1796875000000000000, 0.1875000000000000000, 0.1953125000000000000, 0.2031250000000000000, 0.2109375000000000000, 0.2187500000000000000, 0.2265625000000000000, 0.2343750000000000000, 0.2421875000000000000, 0.2500000000000000000, 0.2578125000000000000, 0.2656250000000000000, 0.2734375000000000000, 0.2812500000000000000, 0.2890625000000000000, 0.2968750000000000000, 0.3046875000000000000, 0.3125000000000000000, 0.3203125000000000000, 0.3281250000000000000, 0.3359375000000000000, 0.3437500000000000000, 0.3515625000000000000, 0.3593750000000000000, 0.3671875000000000000, 0.3750000000000000000, 0.3828125000000000000, 0.3906250000000000000, 0.3984375000000000000, 0.4062500000000000000, 0.4140625000000000000, 0.4218750000000000000, 0.4296875000000000000, 0.4375000000000000000, 0.4453125000000000000, 0.4531250000000000000, 0.4609375000000000000, 0.4687500000000000000, 0.4765625000000000000, 0.4843750000000000000, 0.4921875000000000000, 0.5000000000000000000, 0.5078125000000000000, 0.5156250000000000000, 0.5234375000000000000, 0.5312500000000000000, 0.5390625000000000000, 0.5468750000000000000, 0.5546875000000000000, 0.5625000000000000000, 0.5703125000000000000, 0.5781250000000000000, 0.5859375000000000000, 0.5937500000000000000, 0.6015625000000000000, 0.6093750000000000000, 0.6171875000000000000, 0.6250000000000000000, 0.6328125000000000000, 0.6406250000000000000, 0.6484375000000000000, 0.6562500000000000000, 0.6640625000000000000, 0.6718750000000000000, 0.6796875000000000000, 0.6875000000000000000, 0.6953125000000000000, 0.7031250000000000000, 0.7109375000000000000, 0.7187500000000000000, 0.7265625000000000000, 0.7343750000000000000, 0.7421875000000000000, 0.7500000000000000000, 0.7578125000000000000, 0.7656250000000000000, 0.7734375000000000000, 0.7812500000000000000, 0.7890625000000000000, 0.7968750000000000000, 0.8046875000000000000, 0.8125000000000000000, 0.8203125000000000000, 0.8281250000000000000, 0.8359375000000000000, 0.8437500000000000000, 0.8515625000000000000, 0.8593750000000000000, 0.8671875000000000000, 0.8750000000000000000, 0.8828125000000000000, 0.8906250000000000000, 0.8984375000000000000, 0.9062500000000000000, 0.9140625000000000000, 0.9218750000000000000, 0.9296875000000000000, 0.9375000000000000000, 0.9453125000000000000, 0.9531250000000000000, 0.9609375000000000000, 0.9687500000000000000 ),
 .UNSPECIFIED. ) 
 GEOMETRIC_REPRESENTATION_ITEM ( )  RATIONAL_B_SPLINE_SURFACE ( (
 ( 1.000000000000000000, 0.9238795325112867385, 1.000000000000000000, 0.9238795325112867385, 1.000000000000000000, 0.9238795325112867385, 1.000000000000000000, 0.9238795325112867385, 1.000000000000000000, 0.9238795325112867385, 1.000000000000000000, 0.9238795325112867385, 1.000000000000000000, 0.9238795325112867385, 1.000000000000000000, 0.9238795325112867385, 1.000000000000000000, 0.9238795325112867385, 1.000000000000000000, 0.9238795325112867385, 1.000000000000000000, 0.9238795325112867385, 1.000000000000000000, 0.9238795325112867385, 1.000000000000000000, 0.9238795325112867385, 1.000000000000000000, 0.9238795325112867385, 1.000000000000000000, 0.9238795325112867385, 1.000000000000000000, 0.9238795325112867385, 1.000000000000000000, 0.9238795325112867385, 1.000000000000000000, 0.9238795325112867385, 1.000000000000000000, 0.9238795325112867385, 1.000000000000000000, 0.9238795325112867385, 1.000000000000000000, 0.9238795325112867385, 1.000000000000000000, 0.9238795325112867385, 1.000000000000000000, 0.9238795325112867385, 1.000000000000000000, 0.9238795325112867385, 1.000000000000000000, 0.9238795325112867385, 1.000000000000000000, 0.9238795325112867385, 1.000000000000000000, 0.9238795325112867385, 1.000000000000000000, 0.9238795325112867385, 1.000000000000000000, 0.9238795325112867385, 1.000000000000000000, 0.9238795325112867385, 1.000000000000000000, 0.9238795325112867385, 1.000000000000000000, 0.9238795325112867385, 1.000000000000000000, 0.9238795325112867385, 1.000000000000000000, 0.9238795325112867385, 1.000000000000000000, 0.9238795325112867385, 1.000000000000000000, 0.9238795325112867385, 1.000000000000000000, 0.9238795325112867385, 1.000000000000000000, 0.9238795325112867385, 1.000000000000000000, 0.9238795325112867385, 1.000000000000000000, 0.9238795325112867385, 1.000000000000000000, 0.9238795325112867385, 1.000000000000000000, 0.9238795325112867385, 1.000000000000000000, 0.9238795325112867385, 1.000000000000000000, 0.9238795325112867385, 1.000000000000000000, 0.9238795325112867385, 1.000000000000000000, 0.9238795325112867385, 1.000000000000000000, 0.9238795325112867385, 1.000000000000000000, 0.9238795325112867385, 1.000000000000000000, 0.9238795325112867385, 1.000000000000000000, 0.9238795325112867385, 1.000000000000000000, 0.9238795325112867385, 1.000000000000000000, 0.9238795325112867385, 1.000000000000000000, 0.9238795325112867385, 1.000000000000000000, 0.9238795325112867385, 1.000000000000000000, 0.9238795325112867385, 1.000000000000000000, 0.9238795325112867385, 1.000000000000000000, 0.9238795325112867385, 1.000000000000000000, 0.9238795325112867385, 1.000000000000000000, 0.9238795325112867385, 1.000000000000000000, 0.9238795325112867385, 1.000000000000000000, 0.9238795325112867385, 1.000000000000000000, 0.9238795325112867385, 1.000000000000000000, 0.9238795325112867385, 1.000000000000000000, 0.9238795325112867385, 1.000000000000000000, 0.9238795325112867385, 1.000000000000000000, 0.9238795325112867385, 1.000000000000000000, 0.9238795325112867385, 1.000000000000000000, 0.9238795325112867385, 1.000000000000000000, 0.9238795325112867385, 1.000000000000000000, 0.9238795325112867385, 1.000000000000000000, 0.9238795325112867385, 1.000000000000000000, 0.9238795325112867385, 1.000000000000000000, 0.9238795325112867385, 1.000000000000000000, 0.9238795325112867385, 1.000000000000000000, 0.9238795325112867385, 1.000000000000000000, 0.9238795325112867385, 1.000000000000000000, 0.9238795325112867385, 1.000000000000000000, 0.9238795325112867385, 1.000000000000000000, 0.9238795325112867385, 1.000000000000000000, 0.9238795325112867385, 1.000000000000000000, 0.9238795325112867385, 1.000000000000000000, 0.9238795325112867385, 1.000000000000000000, 0.9238795325112867385, 1.000000000000000000, 0.9238795325112867385, 1.000000000000000000, 0.9238795325112867385, 1.000000000000000000, 0.9238795325112867385, 1.000000000000000000, 0.9238795325112867385, 1.000000000000000000, 0.9238795325112867385, 1.000000000000000000, 0.9238795325112867385, 1.000000000000000000, 0.9238795325112867385, 1.000000000000000000, 0.9238795325112867385, 1.000000000000000000, 0.9238795325112867385, 1.000000000000000000, 0.9238795325112867385, 1.000000000000000000, 0.9238795325112867385, 1.000000000000000000, 0.9238795325112867385, 1.000000000000000000, 0.9238795325112867385, 1.000000000000000000, 0.9238795325112867385, 1.000000000000000000, 0.9238795325112867385, 1.000000000000000000, 0.9238795325112867385, 1.000000000000000000, 0.9238795325112867385, 1.000000000000000000, 0.9238795325112867385, 1.000000000000000000, 0.9238795325112867385, 1.000000000000000000, 0.9238795325112867385, 1.000000000000000000, 0.9238795325112867385, 1.000000000000000000, 0.9238795325112867385, 1.000000000000000000, 0.9238795325112867385, 1.000000000000000000, 0.9238795325112867385, 1.000000000000000000, 0.9238795325112867385, 1.000000000000000000, 0.9238795325112867385, 1.000000000000000000, 0.9238795325112867385, 1.000000000000000000, 0.9238795325112867385, 1.000000000000000000, 0.9238795325112867385, 1.000000000000000000, 0.9238795325112867385, 1.000000000000000000, 0.9238795325112867385, 1.000000000000000000, 0.9238795325112867385, 1.000000000000000000, 0.9238795325112867385, 1.000000000000000000, 0.9238795325112867385, 1.000000000000000000, 0.9238795325112867385, 1.000000000000000000, 0.9238795325112867385, 1.000000000000000000, 0.9238795325112867385, 1.000000000000000000, 0.9238795325112867385, 1.000000000000000000, 0.9238795325112867385, 1.000000000000000000, 0.9238795325112867385, 1.000000000000000000, 0.9238795325112867385, 1.000000000000000000),
 ( 1.000000000000000000, 0.9238795325112867385, 1.000000000000000000, 0.9238795325112867385, 1.000000000000000000, 0.9238795325112867385, 1.000000000000000000, 0.9238795325112867385, 1.000000000000000000, 0.9238795325112867385, 1.000000000000000000, 0.9238795325112867385, 1.000000000000000000, 0.9238795325112867385, 1.000000000000000000, 0.9238795325112867385, 1.000000000000000000, 0.9238795325112867385, 1.000000000000000000, 0.9238795325112867385, 1.000000000000000000, 0.9238795325112867385, 1.000000000000000000, 0.9238795325112867385, 1.000000000000000000, 0.9238795325112867385, 1.000000000000000000, 0.9238795325112867385, 1.000000000000000000, 0.9238795325112867385, 1.000000000000000000, 0.9238795325112867385, 1.000000000000000000, 0.9238795325112867385, 1.000000000000000000, 0.9238795325112867385, 1.000000000000000000, 0.9238795325112867385, 1.000000000000000000, 0.9238795325112867385, 1.000000000000000000, 0.9238795325112867385, 1.000000000000000000, 0.9238795325112867385, 1.000000000000000000, 0.9238795325112867385, 1.000000000000000000, 0.9238795325112867385, 1.000000000000000000, 0.9238795325112867385, 1.000000000000000000, 0.9238795325112867385, 1.000000000000000000, 0.9238795325112867385, 1.000000000000000000, 0.9238795325112867385, 1.000000000000000000, 0.9238795325112867385, 1.000000000000000000, 0.9238795325112867385, 1.000000000000000000, 0.9238795325112867385, 1.000000000000000000, 0.9238795325112867385, 1.000000000000000000, 0.9238795325112867385, 1.000000000000000000, 0.9238795325112867385, 1.000000000000000000, 0.9238795325112867385, 1.000000000000000000, 0.9238795325112867385, 1.000000000000000000, 0.9238795325112867385, 1.000000000000000000, 0.9238795325112867385, 1.000000000000000000, 0.9238795325112867385, 1.000000000000000000, 0.9238795325112867385, 1.000000000000000000, 0.9238795325112867385, 1.000000000000000000, 0.9238795325112867385, 1.000000000000000000, 0.9238795325112867385, 1.000000000000000000, 0.9238795325112867385, 1.000000000000000000, 0.9238795325112867385, 1.000000000000000000, 0.9238795325112867385, 1.000000000000000000, 0.9238795325112867385, 1.000000000000000000, 0.9238795325112867385, 1.000000000000000000, 0.9238795325112867385, 1.000000000000000000, 0.9238795325112867385, 1.000000000000000000, 0.9238795325112867385, 1.000000000000000000, 0.9238795325112867385, 1.000000000000000000, 0.9238795325112867385, 1.000000000000000000, 0.9238795325112867385, 1.000000000000000000, 0.9238795325112867385, 1.000000000000000000, 0.9238795325112867385, 1.000000000000000000, 0.9238795325112867385, 1.000000000000000000, 0.9238795325112867385, 1.000000000000000000, 0.9238795325112867385, 1.000000000000000000, 0.9238795325112867385, 1.000000000000000000, 0.9238795325112867385, 1.000000000000000000, 0.9238795325112867385, 1.000000000000000000, 0.9238795325112867385, 1.000000000000000000, 0.9238795325112867385, 1.000000000000000000, 0.9238795325112867385, 1.000000000000000000, 0.9238795325112867385, 1.000000000000000000, 0.9238795325112867385, 1.000000000000000000, 0.9238795325112867385, 1.000000000000000000, 0.9238795325112867385, 1.000000000000000000, 0.9238795325112867385, 1.000000000000000000, 0.9238795325112867385, 1.000000000000000000, 0.9238795325112867385, 1.000000000000000000, 0.9238795325112867385, 1.000000000000000000, 0.9238795325112867385, 1.000000000000000000, 0.9238795325112867385, 1.000000000000000000, 0.9238795325112867385, 1.000000000000000000, 0.9238795325112867385, 1.000000000000000000, 0.9238795325112867385, 1.000000000000000000, 0.9238795325112867385, 1.000000000000000000, 0.9238795325112867385, 1.000000000000000000, 0.9238795325112867385, 1.000000000000000000, 0.9238795325112867385, 1.000000000000000000, 0.9238795325112867385, 1.000000000000000000, 0.9238795325112867385, 1.000000000000000000, 0.9238795325112867385, 1.000000000000000000, 0.9238795325112867385, 1.000000000000000000, 0.9238795325112867385, 1.000000000000000000, 0.9238795325112867385, 1.000000000000000000, 0.9238795325112867385, 1.000000000000000000, 0.9238795325112867385, 1.000000000000000000, 0.9238795325112867385, 1.000000000000000000, 0.9238795325112867385, 1.000000000000000000, 0.9238795325112867385, 1.000000000000000000, 0.9238795325112867385, 1.000000000000000000, 0.9238795325112867385, 1.000000000000000000, 0.9238795325112867385, 1.000000000000000000, 0.9238795325112867385, 1.000000000000000000, 0.9238795325112867385, 1.000000000000000000, 0.9238795325112867385, 1.000000000000000000, 0.9238795325112867385, 1.000000000000000000, 0.9238795325112867385, 1.000000000000000000, 0.9238795325112867385, 1.000000000000000000, 0.9238795325112867385, 1.000000000000000000, 0.9238795325112867385, 1.000000000000000000, 0.9238795325112867385, 1.000000000000000000, 0.9238795325112867385, 1.000000000000000000, 0.9238795325112867385, 1.000000000000000000, 0.9238795325112867385, 1.000000000000000000, 0.9238795325112867385, 1.000000000000000000, 0.9238795325112867385, 1.000000000000000000, 0.9238795325112867385, 1.000000000000000000, 0.9238795325112867385, 1.000000000000000000, 0.9238795325112867385, 1.000000000000000000, 0.9238795325112867385, 1.000000000000000000, 0.9238795325112867385, 1.000000000000000000, 0.9238795325112867385, 1.000000000000000000, 0.9238795325112867385, 1.000000000000000000, 0.9238795325112867385, 1.000000000000000000, 0.9238795325112867385, 1.000000000000000000, 0.9238795325112867385, 1.000000000000000000, 0.9238795325112867385, 1.000000000000000000, 0.9238795325112867385, 1.000000000000000000, 0.9238795325112867385, 1.000000000000000000, 0.9238795325112867385, 1.000000000000000000) ) ) 
 REPRESENTATION_ITEM ( '' )  SURFACE ( )  );
#3019=CARTESIAN_POINT ( 'NONE',  ( 16.81250000000011013, -2.649519052838178457, 1.097466725451499370 ) ) ;
#3035=CYLINDRICAL_SURFACE ( 'NONE', #15215, 2.499999999999999112 ) ;
#3038=CARTESIAN_POINT ( 'NONE',  ( 23.43750000000010303, -1.999999999999851674, 0.8284271247462955401 ) ) ;
#3045=CARTESIAN_POINT ( 'NONE',  ( 17.75000000000018119, 1.873492889145067508, 1.873492889144734441 ) ) ;
#3054=ORIENTED_EDGE ( 'NONE', *, *, #9514, .T. ) ;
#3064=CARTESIAN_POINT ( 'NONE',  ( 15.06250000000016165, 2.000000000000151879, 0.8284271247461152399 ) ) ;
#3065=EDGE_CURVE ( 'NONE', #23806, #13194, #27318, .T. ) ;
#3117=CARTESIAN_POINT ( 'NONE',  ( 13.75000000000006750, 2.220446049250313081E-13, -2.000000000000001776 ) ) ;
#3126=CARTESIAN_POINT ( 'NONE',  ( 16.50000000000004263, -1.999999999999835243, 0.000000000000000000 ) ) ;
#3132=CYLINDRICAL_SURFACE ( 'NONE', #531, 2.499999999999999112 ) ;
#3146=CARTESIAN_POINT ( 'NONE',  ( 9.500000000000092371, 1.873492889145067508, -1.873492889145011997 ) ) ;
#3160=ORIENTED_EDGE ( 'NONE', *, *, #14682, .F. ) ;
#3162=CARTESIAN_POINT ( 'NONE',  ( 20.43750000000011369, 2.649519052838478661, 1.097466725451499370 ) ) ;
#3181=CARTESIAN_POINT ( 'NONE',  ( 24.06250000000009592, 2.000000000000091926, 0.8284271247461153509 ) ) ;
#3194=CARTESIAN_POINT ( 'NONE',  ( 24.77698899409918809, 1.864818660053481736, -1.235634622128368942 ) ) ;
#3199=AXIS2_PLACEMENT_3D ( 'NONE', #29275, #3623, #6098 ) ;
#3202=CARTESIAN_POINT ( 'NONE',  ( 19.08632486540534501, -1.767766952966154381, 1.767766952966376426 ) ) ;
#3204=CARTESIAN_POINT ( 'NONE',  ( 17.18750000000013145, 0.8284271247463557142, 1.999999999999971800 ) ) ;
#3225=CARTESIAN_POINT ( 'NONE',  ( 10.62500000000013500, -1.414213562372979016, -1.414213562373090038 ) ) ;
#3230=CARTESIAN_POINT ( 'NONE',  ( 11.46132486540535389, 1.110223024625156540E-13, -2.500000000000002220 ) ) ;
#3234=CARTESIAN_POINT ( 'NONE',  ( 10.18750000000014033, 0.8284271247463557142, 2.000000000000031530 ) ) ;
#3260=CARTESIAN_POINT ( 'NONE',  ( 15.37500000000011013, -1.414213562373034527, 1.414213562373034527 ) ) ;
#3273=CARTESIAN_POINT ( 'NONE',  ( 17.81250000000015632, 0.8284271247463557142, -2.000000000000091926 ) ) ;
#3277=CARTESIAN_POINT ( 'NONE',  ( 13.18750000000012967, 1.097466725451619718, -2.649519052838358757 ) ) ;
#3280=VECTOR ( 'NONE', #15350, 1000.000000000000000 ) ;
#3328=CARTESIAN_POINT ( 'NONE',  ( 23.31250000000007461, -0.8284271247460553989, 2.000000000000091926 ) ) ;
#3336=CARTESIAN_POINT ( 'NONE',  ( 15.75000000000006928, 1.873492889145123019, 1.873492889144734441 ) ) ;
#3353=CARTESIAN_POINT ( 'NONE',  ( 14.25000000000012434, 5.551115123125782702E-14, 2.000000000000001776 ) ) ;
#3356=( BOUNDED_CURVE ( )  B_SPLINE_CURVE ( 2, ( #17551, #22755, #26869, #1385, #5830, #10795, #29492, #6154, #23371 ),
 .UNSPECIFIED., .F., .T. ) 
 B_SPLINE_CURVE_WITH_KNOTS ( ( 3, 2, 2, 2, 3 ),
 ( 0.4843750000000000000, 0.4921875000000000000, 0.5000000000000000000, 0.5078125000000000000, 0.5156250000000000000 ),
 .UNSPECIFIED. ) 
 CURVE ( )  GEOMETRIC_REPRESENTATION_ITEM ( )  RATIONAL_B_SPLINE_CURVE ( ( 1.000000000000000000, 0.9238795325112867385, 1.000000000000000000, 0.9238795325112867385, 1.000000000000000000, 0.9238795325112867385, 1.000000000000000000, 0.9238795325112867385, 1.000000000000000000 ) ) 
 REPRESENTATION_ITEM ( '' )  );
#3359=CARTESIAN_POINT ( 'NONE',  ( 13.72617513459485927, -2.499999999999904521, 1.035533905932689347 ) ) ;
#3368=ORIENTED_EDGE ( 'NONE', *, *, #20291, .T. ) ;
#3379=CARTESIAN_POINT ( 'NONE',  ( 11.25000000000001066, 1.110223024625156540E-13, 1.999999999999946265 ) ) ;
#3412=CARTESIAN_POINT ( 'NONE',  ( 14.00000000000006750, 2.000000000000112799, 0.000000000000000000 ) ) ;
#3419=CARTESIAN_POINT ( 'NONE',  ( 17.43750000000013145, -1.999999999999851674, 0.8284271247463557142 ) ) ;
#3430=EDGE_CURVE ( 'NONE', #19618, #27870, #8492, .T. ) ;
#3431=EDGE_CURVE ( 'NONE', #4040, #1574, #22411, .T. ) ;
#3448=DIRECTION ( 'NONE',  ( -1.000000000000000000, -1.665334536937731113E-16, 1.526556658859586792E-16 ) ) ;
#3452=CARTESIAN_POINT ( 'NONE',  ( 24.89327801240793647, 1.031043948637415886, -1.842165862623910799 ) ) ;
#3486=CARTESIAN_POINT ( 'NONE',  ( 14.87500000000002665, 1.665334536937734811E-13, 2.649519052838278377 ) ) ;
#3501=ADVANCED_FACE ( 'NONE', ( #28794 ), #5297, .T. ) ;
#3511=CARTESIAN_POINT ( 'NONE',  ( 17.25000000000001421, 1.665334536937734811E-13, 2.000000000000001776 ) ) ;
#3540=CARTESIAN_POINT ( 'NONE',  ( 9.750000000000119016, 1.665334536937734811E-13, -1.999999999999890754 ) ) ;
#3543=CARTESIAN_POINT ( 'NONE',  ( 24.93750000000011013, 2.000000000000151879, -0.8284271247462354770 ) ) ;
#3554=MECHANICAL_DESIGN_GEOMETRIC_PRESENTATION_REPRESENTATION('',(#30058),#10480);
#3557=CARTESIAN_POINT ( 'NONE',  ( 16.47617513459488237, 1.035533905932929599, 2.499999999999844569 ) ) ;
#3562=VERTEX_POINT ( 'NONE', #5446 ) ;
#3576=CARTESIAN_POINT ( 'NONE',  ( 16.25000000000009948, 1.665334536937734811E-13, 2.000000000000001776 ) ) ;
#3580=CARTESIAN_POINT ( 'NONE',  ( 13.12500000000013678, 1.665334536937734811E-13, -2.649519052838444910 ) ) ;
#3623=DIRECTION ( 'NONE',  ( -1.000000000000000000, -1.665334536937731113E-16, 1.526556658859586792E-16 ) ) ;
#3624=DIRECTION ( 'NONE',  ( -1.000000000000000000, -1.665334536937731113E-16, 1.526556658859586792E-16 ) ) ;
#3637=CARTESIAN_POINT ( 'NONE',  ( 14.00000000000020606, -1.873492889144789952, 1.873492889144956486 ) ) ;
#3661=CARTESIAN_POINT ( 'NONE',  ( 15.87500000000008349, 1.414213562373201061, -1.414213562373090038 ) ) ;
#3666=CARTESIAN_POINT ( 'NONE',  ( 13.97617513459482730, -1.035533905932629173, -2.499999999999904521 ) ) ;
#3688=CARTESIAN_POINT ( 'NONE',  ( 19.66367513459493921, -1.767766952966209892, 1.767766952966376426 ) ) ;
#3712=CARTESIAN_POINT ( 'NONE',  ( 16.22617513459482552, 2.500000000000144773, -1.035533905932869425 ) ) ;
#3733=CARTESIAN_POINT ( 'NONE',  ( 18.81250000000011013, 0.8284271247462354770, -2.000000000000091926 ) ) ;
#3737=CARTESIAN_POINT ( 'NONE',  ( 13.68750000000000178, -1.097466725451499370, 2.649519052838178457 ) ) ;
#3748=CARTESIAN_POINT ( 'NONE',  ( 19.77382486540529172, 2.500000000000144773, 1.035533905932629173 ) ) ;
#3749=VECTOR ( 'NONE', #22160, 1000.000000000000000 ) ;
#3750=PRODUCT_DEFINITION_SHAPE ( 'NONE', 'NONE',  #21369 ) ;
#3761=CARTESIAN_POINT ( 'NONE',  ( 21.81250000000009592, 0.8284271247462955401, -2.000000000000151879 ) ) ;
#3789=CARTESIAN_POINT ( 'NONE',  ( 13.22617513459483618, 2.500000000000024425, -1.035533905932929599 ) ) ;
#3794=CARTESIAN_POINT ( 'NONE',  ( 14.62500000000013856, 2.649519052838555933, 1.110223024625156540E-13 ) ) ;
#3822=CARTESIAN_POINT ( 'NONE',  ( 13.60117513459492145, -1.035533905932689347, 2.499999999999904521 ) ) ;
#3835=CARTESIAN_POINT ( 'NONE',  ( 23.81250000000009948, 1.097466725451619718, 2.649519052838298805 ) ) ;
#3842=CARTESIAN_POINT ( 'NONE',  ( 10.00000000000014921, 2.023458278065096039, 0.3436007916004408802 ) ) ;
#3846=ORIENTED_EDGE ( 'NONE', *, *, #809, .T. ) ;
#3851=CARTESIAN_POINT ( 'NONE',  ( 22.43750000000002842, -1.999999999999851674, 0.8284271247462354770 ) ) ;
#3852=CARTESIAN_POINT ( 'NONE',  ( 0.000000000000000000, 0.000000000000000000, 0.000000000000000000 ) ) ;
#3857=CARTESIAN_POINT ( 'NONE',  ( 12.41367513459484861, 1.767766952966431937, 1.767766952966209892 ) ) ;
#3870=ORIENTED_EDGE ( 'NONE', *, *, #30228, .F. ) ;
#3880=CARTESIAN_POINT ( 'NONE',  ( 12.50000000000012257, -1.999999999999835243, 0.000000000000000000 ) ) ;
#3912=FACE_OUTER_BOUND ( 'NONE', #18123, .T. ) ;
#3913=CARTESIAN_POINT ( 'NONE',  ( 24.86659270085223739, 0.5400564011831616718, -2.082004388006507778 ) ) ;
#3932=CARTESIAN_POINT ( 'NONE',  ( 23.71132486540528106, 2.500000000000168754, -1.110223024625156540E-13 ) ) ;
#3938=CARTESIAN_POINT ( 'NONE',  ( 15.06250000000013323, -2.649519052838178457, 1.097466725451439196 ) ) ;
#3965=CARTESIAN_POINT ( 'NONE',  ( 20.39882486540528816, -1.035533905932689347, -2.499999999999904521 ) ) ;
#3968=CARTESIAN_POINT ( 'NONE',  ( 11.25000000000001066, 1.110223024625156540E-13, 1.999999999999946265 ) ) ;
#3983=ORIENTED_EDGE ( 'NONE', *, *, #3430, .F. ) ;
#3992=CARTESIAN_POINT ( 'NONE',  ( 9.875000000000023093, 1.414213562373201061, -1.414213562373090038 ) ) ;
#4002=MANIFOLD_SOLID_BREP ( 'Cut-Sweep1', #29107 ) ;
#4005=ORIENTED_EDGE ( 'NONE', *, *, #16747, .T. ) ;
#4007=VECTOR ( 'NONE', #11154, 1000.000000000000000 ) ;
#4009=CARTESIAN_POINT ( 'NONE',  ( 22.18750000000018119, 0.8284271247464156662, 1.999999999999971800 ) ) ;
#4017=CARTESIAN_POINT ( 'NONE',  ( 16.53867513459489302, 5.551115123125782702E-14, 2.500000000000002220 ) ) ;
#4020=CARTESIAN_POINT ( 'NONE',  ( 16.53867513459489302, 5.551115123125782702E-14, 2.500000000000002220 ) ) ;
#4021=EDGE_LOOP ( 'NONE', ( #21601, #2613, #13305 ) ) ;
#4039=CARTESIAN_POINT ( 'NONE',  ( 12.43750000000010836, -1.999999999999851674, 0.8284271247462955401 ) ) ;
#4040=VERTEX_POINT ( 'NONE', #20644 ) ;
#4051=LINE ( 'NONE', #22973, #4007 ) ;
#4062=CARTESIAN_POINT ( 'NONE',  ( 20.06250000000006395, 2.000000000000151879, 0.8284271247461753029 ) ) ;
#4102=CARTESIAN_POINT ( 'NONE',  ( 11.93750000000005507, -1.097466725451379244, 2.649519052838238409 ) ) ;
#4107=ORIENTED_EDGE ( 'NONE', *, *, #6430, .F. ) ;
#4116=CARTESIAN_POINT ( 'NONE',  ( 10.31249999999998934, -0.8284271247461753029, 1.999999999999911626 ) ) ;
#4125=CARTESIAN_POINT ( 'NONE',  ( 12.62500000000013678, -1.414213562372979016, -1.414213562373145550 ) ) ;
#4129=DIRECTION ( 'NONE',  ( -1.000000000000000000, -1.665334536937731113E-16, 1.526556658859586792E-16 ) ) ;
#4143=DIRECTION ( 'NONE',  ( -1.000000000000000000, -1.665334536937731113E-16, 1.526556658859586792E-16 ) ) ;
#4160=CARTESIAN_POINT ( 'NONE',  ( 21.37500000000011724, -1.414213562373090038, 1.414213562373034527 ) ) ;
#4178=ORIENTED_EDGE ( 'NONE', *, *, #24090, .F. ) ;
#4181=DIRECTION ( 'NONE',  ( -1.000000000000000000, -1.665334536937731113E-16, 1.526556658859586792E-16 ) ) ;
#4184=( BOUNDED_CURVE ( )  B_SPLINE_CURVE ( 2, ( #30004, #8978, #1746, #8830, #27841, #25549, #25389, #29697, #4347 ),
 .UNSPECIFIED., .F., .T. ) 
 B_SPLINE_CURVE_WITH_KNOTS ( ( 3, 2, 2, 2, 3 ),
 ( 0.5156250000000000000, 0.5234375000000000000, 0.5312500000000000000, 0.5390625000000000000, 0.5468750000000000000 ),
 .UNSPECIFIED. ) 
 CURVE ( )  GEOMETRIC_REPRESENTATION_ITEM ( )  RATIONAL_B_SPLINE_CURVE ( ( 1.000000000000000000, 0.9238795325112867385, 1.000000000000000000, 0.9238795325112867385, 1.000000000000000000, 0.9238795325112867385, 1.000000000000000000, 0.9238795325112867385, 1.000000000000000000 ) ) 
 REPRESENTATION_ITEM ( '' )  );
#4190=CARTESIAN_POINT ( 'NONE',  ( 13.00000000000003908, 2.000000000000112799, 0.000000000000000000 ) ) ;
#4195=CARTESIAN_POINT ( 'NONE',  ( 12.68750000000013678, -0.8284271247459952248, -1.999999999999911626 ) ) ;
#4198=ORIENTED_EDGE ( 'NONE', *, *, #12094, .T. ) ;
#4215=ADVANCED_FACE ( 'NONE', ( #223 ), #19133, .T. ) ;
#4221=CARTESIAN_POINT ( 'NONE',  ( 18.31249999999999289, -0.8284271247460552878, 2.000000000000031530 ) ) ;
#4240=EDGE_LOOP ( 'NONE', ( #16191, #3054, #29890, #30048 ) ) ;
#4248=CARTESIAN_POINT ( 'NONE',  ( 21.33632486540526685, -1.767766952966265404, -1.767766952966487448 ) ) ;
#4252=DIRECTION ( 'NONE',  ( -1.000000000000000000, -1.665334536937731113E-16, 1.526556658859586792E-16 ) ) ;
#4256=CARTESIAN_POINT ( 'NONE',  ( 12.50000000000009415, 1.873492889145011997, -1.873492889144900975 ) ) ;
#4258=CARTESIAN_POINT ( 'NONE',  ( 12.64882486540515671, 2.500000000000084821, -1.035533905932929599 ) ) ;
#4274=CARTESIAN_POINT ( 'NONE',  ( 21.68750000000009592, -1.097466725451439196, 2.649519052838298805 ) ) ;
#4284=CARTESIAN_POINT ( 'NONE',  ( 13.31250000000012612, -0.8284271247460552878, 1.999999999999911626 ) ) ;
#4311=CARTESIAN_POINT ( 'NONE',  ( 17.27382486540533080, -2.499999999999844569, -1.035533905932809473 ) ) ;
#4315=CARTESIAN_POINT ( 'NONE',  ( 21.64882486540524553, 2.500000000000084821, -1.035533905932929599 ) ) ;
#4322=CARTESIAN_POINT ( 'NONE',  ( 23.75000000000013145, 1.665334536937734811E-13, -2.000000000000057288 ) ) ;
#4344=CARTESIAN_POINT ( 'NONE',  ( 13.12500000000016342, 1.414213562373145550, 1.414213562373034527 ) ) ;
#4347=CARTESIAN_POINT ( 'NONE',  ( 18.53867513459497829, 1.665334536937734811E-13, 2.499999999999946709 ) ) ;
#4351=CARTESIAN_POINT ( 'NONE',  ( 10.18750000000014033, 0.8284271247463557142, 2.000000000000031530 ) ) ;
#4359=CARTESIAN_POINT ( 'NONE',  ( 19.53867513459495342, 5.551115123125782702E-14, 2.500000000000002220 ) ) ;
#4377=PLANE ( 'NONE',  #7230 ) ;
#4395=CONICAL_SURFACE ( 'NONE', #24975, 2.499999999999999112, 0.7853981633974522758 ) ;
#4408=CARTESIAN_POINT ( 'NONE',  ( 11.37500000000007994, 2.220446049250313081E-13, -2.649519052838444910 ) ) ;
#4420=AXIS2_PLACEMENT_3D ( 'NONE', #10080, #6055, #981 ) ;
#4421=ORIENTED_EDGE ( 'NONE', *, *, #4778, .F. ) ;
#4425=CARTESIAN_POINT ( 'NONE',  ( 21.87500000000008882, -2.649519052838111843, 1.110223024625156540E-13 ) ) ;
#4434=CARTESIAN_POINT ( 'NONE',  ( 12.81250000000004441, 0.8284271247461753029, -2.000000000000091926 ) ) ;
#4452=CARTESIAN_POINT ( 'NONE',  ( 21.87500000000006040, 1.110223024625156540E-13, 2.649519052838167354 ) ) ;
#4464=CARTESIAN_POINT ( 'NONE',  ( 10.00000000000014744, 0.5735884529305894652, 2.302716324837206230 ) ) ;
#4472=CARTESIAN_POINT ( 'NONE',  ( 14.97617513459490191, -1.035533905932568999, -2.499999999999904521 ) ) ;
#4473=CARTESIAN_POINT ( 'NONE',  ( 21.50000000000004619, -1.999999999999890754, -1.665334536937734811E-13 ) ) ;
#4481=VECTOR ( 'NONE', #29362, 1000.000000000000000 ) ;
#4482=CARTESIAN_POINT ( 'NONE',  ( 24.67146418439117639, -2.317096007398430579, 0.2759497617555390914 ) ) ;
#4508=CARTESIAN_POINT ( 'NONE',  ( 11.62499999999999645, -1.414213562373090038, -1.414213562373090038 ) ) ;
#4511=CARTESIAN_POINT ( 'NONE',  ( 10.00000000000015099, 1.032209696753886519, -2.067976829748041645 ) ) ;
#4532=CARTESIAN_POINT ( 'NONE',  ( 20.43750000000014566, -1.999999999999911626, 0.8284271247462354770 ) ) ;
#4543=( BOUNDED_CURVE ( )  B_SPLINE_CURVE ( 2, ( #28951, #14860, #16886, #28800, #21322, #17027, #14571, #12282, #12135 ),
 .UNSPECIFIED., .F., .T. ) 
 B_SPLINE_CURVE_WITH_KNOTS ( ( 3, 2, 2, 2, 3 ),
 ( 0.6406250000000000000, 0.6484375000000000000, 0.6562500000000000000, 0.6640625000000000000, 0.6718750000000000000 ),
 .UNSPECIFIED. ) 
 CURVE ( )  GEOMETRIC_REPRESENTATION_ITEM ( )  RATIONAL_B_SPLINE_CURVE ( ( 1.000000000000000000, 0.9238795325112867385, 1.000000000000000000, 0.9238795325112867385, 1.000000000000000000, 0.9238795325112867385, 1.000000000000000000, 0.9238795325112867385, 1.000000000000000000 ) ) 
 REPRESENTATION_ITEM ( '' )  );
#4567=CARTESIAN_POINT ( 'NONE',  ( 11.87500000000013500, 1.665334536937734811E-13, 2.649519052838278377 ) ) ;
#4569=CARTESIAN_POINT ( 'NONE',  ( 12.96132486540529882, 1.110223024625156540E-13, 2.500000000000002220 ) ) ;
#4572=CARTESIAN_POINT ( 'NONE',  ( 23.97617513459492145, -1.035533905932689347, -2.500000000000084821 ) ) ;
#4580=CARTESIAN_POINT ( 'NONE',  ( 20.87500000000011724, -2.649519052838167354, -5.551115123125782702E-14 ) ) ;
#4587=CARTESIAN_POINT ( 'NONE',  ( 10.75000000000014921, 1.665334536937734811E-13, -2.000000000000168310 ) ) ;
#4602=CARTESIAN_POINT ( 'NONE',  ( 19.68750000000012790, 2.649519052838478661, 1.097466725451439196 ) ) ;
#4610=CARTESIAN_POINT ( 'NONE',  ( 19.97617513459498539, -1.035533905932629173, -2.499999999999964473 ) ) ;
#4618=CARTESIAN_POINT ( 'NONE',  ( 12.62500000000005329, 1.110223024625156540E-13, 2.649519052838056332 ) ) ;
#4620=CARTESIAN_POINT ( 'NONE',  ( 19.25000000000009948, 1.110223024625156540E-13, 1.999999999999946265 ) ) ;
#4624=CARTESIAN_POINT ( 'NONE',  ( 12.66367513459487526, -1.767766952966265404, 1.767766952966431937 ) ) ;
#4626=CARTESIAN_POINT ( 'NONE',  ( 24.74512076645466152, -1.864212315884203441, -1.303982556562485851 ) ) ;
#4627=CYLINDRICAL_SURFACE ( 'NONE', #27269, 2.499999999999999112 ) ;
#4643=CARTESIAN_POINT ( 'NONE',  ( 11.56250000000009059, -1.999999999999851674, -0.8284271247462354770 ) ) ;
#4674=CARTESIAN_POINT ( 'NONE',  ( 21.18750000000019540, 0.8284271247462955401, 2.000000000000031530 ) ) ;
#4681=ORIENTED_EDGE ( 'NONE', *, *, #262, .F. ) ;
#4684=CARTESIAN_POINT ( 'NONE',  ( 11.64882486540532014, 2.500000000000144773, -1.035533905932809473 ) ) ;
#4712=CARTESIAN_POINT ( 'NONE',  ( 12.56250000000004619, 2.649519052838298805, -1.097466725451739622 ) ) ;
#4731=CARTESIAN_POINT ( 'NONE',  ( 23.75000000000015987, -1.873492889144845464, 1.873492889144900975 ) ) ;
#4738=VECTOR ( 'NONE', #14636, 1000.000000000000000 ) ;
#4753=CARTESIAN_POINT ( 'NONE',  ( 22.06250000000015632, -2.649519052838238409, 1.097466725451559322 ) ) ;
#4761=CARTESIAN_POINT ( 'NONE',  ( 17.39882486540526685, -1.035533905932749299, -2.499999999999964473 ) ) ;
#4764=MECHANICAL_DESIGN_GEOMETRIC_PRESENTATION_REPRESENTATION('',(#28299),#30267);
#4765=ORIENTED_EDGE ( 'NONE', *, *, #19178, .F. ) ;
#4772=CARTESIAN_POINT ( 'NONE',  ( 10.50000000000012079, 1.873492889145123019, 1.873492889144845464 ) ) ;
#4775=CARTESIAN_POINT ( 'NONE',  ( 20.12500000000011369, 1.414213562373201061, 1.414213562373034527 ) ) ;
#4778=EDGE_CURVE ( 'NONE', #6046, #21961, #16371, .T. ) ;
#4783=CARTESIAN_POINT ( 'NONE',  ( 24.84150635094622572, -1.291286745249641628E-13, -2.158493649053927044 ) ) ;
#4786=CARTESIAN_POINT ( 'NONE',  ( 14.47617513459494099, 1.035533905932809473, 2.500000000000024425 ) ) ;
#4821=CARTESIAN_POINT ( 'NONE',  ( 13.27382486540526862, -2.499999999999904521, -1.035533905932749299 ) ) ;
#4828=CARTESIAN_POINT ( 'NONE',  ( 17.00000000000015277, 2.000000000000112799, 0.000000000000000000 ) ) ;
#4840=CARTESIAN_POINT ( 'NONE',  ( 21.18750000000019540, 0.8284271247462955401, 2.000000000000031530 ) ) ;
#4854=CARTESIAN_POINT ( 'NONE',  ( 21.21132486540527751, -2.499999999999891198, -2.220446049250313081E-13 ) ) ;
#4860=CARTESIAN_POINT ( 'NONE',  ( 24.93750000000011013, 2.000000000000151879, -0.8284271247462354770 ) ) ;
#4865=VERTEX_POINT ( 'NONE', #30304 ) ;
#4866=CARTESIAN_POINT ( 'NONE',  ( 15.33632486540528816, -1.767766952966265404, -1.767766952966487448 ) ) ;
#4874=CARTESIAN_POINT ( 'NONE',  ( 21.50000000000010303, 1.873492889145067508, 1.873492889144734441 ) ) ;
#4903=CARTESIAN_POINT ( 'NONE',  ( 17.22617513459484329, 2.500000000000144773, -1.035533905932689347 ) ) ;
#4909=ORIENTED_EDGE ( 'NONE', *, *, #19252, .F. ) ;
#4916=CARTESIAN_POINT ( 'NONE',  ( 18.37500000000008527, -1.414213562373090038, 1.414213562372867994 ) ) ;
#4933=DIRECTION ( 'NONE',  ( -1.000000000000000000, -1.665334536937731113E-16, 1.526556658859586792E-16 ) ) ;
#4971=CARTESIAN_POINT ( 'NONE',  ( 18.18750000000005684, 0.8284271247463557142, 1.999999999999971800 ) ) ;
#4982=CARTESIAN_POINT ( 'NONE',  ( 19.43750000000012790, -1.999999999999851674, 0.8284271247462354770 ) ) ;
#5003=CARTESIAN_POINT ( 'NONE',  ( 9.625000000000106581, 2.649519052838444910, 0.000000000000000000 ) ) ;
#5007=DIRECTION ( 'NONE',  ( -1.000000000000000000, -1.665334536937731113E-16, 1.526556658859586792E-16 ) ) ;
#5017=CARTESIAN_POINT ( 'NONE',  ( 17.50000000000012790, 1.873492889145011997, 1.873492889144734441 ) ) ;
#5025=ORIENTED_EDGE ( 'NONE', *, *, #262, .T. ) ;
#5056=CARTESIAN_POINT ( 'NONE',  ( 11.06250000000006928, 2.000000000000091926, 0.8284271247461753029 ) ) ;
#5059=CARTESIAN_POINT ( 'NONE',  ( 24.46132486540536632, 1.665334536937734811E-13, -2.500000000000002220 ) ) ;
#5060=CARTESIAN_POINT ( 'NONE',  ( 10.31249999999998934, 2.649519052838478661, -1.097466725451679892 ) ) ;
#5064=CARTESIAN_POINT ( 'NONE',  ( 19.50000000000009948, -1.999999999999835243, 0.000000000000000000 ) ) ;
#5067=( BOUNDED_CURVE ( )  B_SPLINE_CURVE ( 2, ( #28499, #7465, #21617, #16876, #26196, #10247, #22523, #27099, #29400 ),
 .UNSPECIFIED., .F., .T. ) 
 B_SPLINE_CURVE_WITH_KNOTS ( ( 3, 2, 2, 2, 3 ),
 ( 0.8906250000000000000, 0.8984375000000000000, 0.9062500000000000000, 0.9140625000000000000, 0.9194088329325865727 ),
 .UNSPECIFIED. ) 
 CURVE ( )  GEOMETRIC_REPRESENTATION_ITEM ( )  RATIONAL_B_SPLINE_CURVE ( ( 1.000000000000000000, 0.9238795325112867385, 1.000000000000000000, 0.9238795325112867385, 1.000000000000000000, 0.9238795325112867385, 1.000000000000000000, 0.9479084336411144340, 0.9671125746062680939 ) ) 
 REPRESENTATION_ITEM ( '' )  );
#5071=( NAMED_UNIT ( * ) PLANE_ANGLE_UNIT ( ) SI_UNIT ( $, .RADIAN. ) );
#5088=EDGE_CURVE ( 'NONE', #25453, #4865, #16960, .T. ) ;
#5089=EDGE_LOOP ( 'NONE', ( #16116, #2289, #8621, #29497 ) ) ;
#5092=EDGE_CURVE ( 'NONE', #13146, #6031, #27490, .T. ) ;
#5119=ORIENTED_EDGE ( 'NONE', *, *, #10938, .F. ) ;
#5126=CARTESIAN_POINT ( 'NONE',  ( 19.93750000000015277, 2.000000000000091926, -0.8284271247462354770 ) ) ;
#5131=( GEOMETRIC_REPRESENTATION_CONTEXT ( 3 ) GLOBAL_UNCERTAINTY_ASSIGNED_CONTEXT ( ( #1314 ) ) GLOBAL_UNIT_ASSIGNED_CONTEXT ( ( #17406, #14508, #2786 ) ) REPRESENTATION_CONTEXT ( 'NONE', 'WORKASPACE' ) );
#5141=EDGE_CURVE ( 'NONE', #6464, #6046, #26332, .T. ) ;
#5153=CARTESIAN_POINT ( 'NONE',  ( 23.81250000000003553, 0.8284271247463557142, -2.000000000000151879 ) ) ;
#5169=CARTESIAN_POINT ( 'NONE',  ( 19.43750000000013145, 2.649519052838358757, 1.097466725451499370 ) ) ;
#5193=CARTESIAN_POINT ( 'NONE',  ( 16.14882486540525619, -2.499999999999904521, 1.035533905932749299 ) ) ;
#5199=ORIENTED_EDGE ( 'NONE', *, *, #6999, .F. ) ;
#5212=CARTESIAN_POINT ( 'NONE',  ( 24.27382486540532369, -2.499999999999904521, -1.035533905932809473 ) ) ;
#5213=CARTESIAN_POINT ( 'NONE',  ( 12.25000000000009415, 1.873492889145123019, -1.873492889144956486 ) ) ;
#5215=ORIENTED_EDGE ( 'NONE', *, *, #3431, .T. ) ;
#5216=CARTESIAN_POINT ( 'NONE',  ( 20.68750000000011369, -0.8284271247459952248, -1.999999999999971800 ) ) ;
#5218=DIRECTION ( 'NONE',  ( -0.7071067811865455743, -1.324765512014429388E-16, 0.7071067811865495711 ) ) ;
#5222=CARTESIAN_POINT ( 'NONE',  ( 2.081668171172167281E-16, 3.582034040661430693E-16, -2.499999999999999112 ) ) ;
#5235=CARTESIAN_POINT ( 'NONE',  ( 11.68750000000000000, -0.8284271247461753029, -1.999999999999971800 ) ) ;
#5238=CARTESIAN_POINT ( 'NONE',  ( 11.33632486540525619, -1.767766952966209892, -1.767766952966598470 ) ) ;
#5246=EDGE_CURVE ( 'NONE', #5319, #13146, #14622, .T. ) ;
#5281=CARTESIAN_POINT ( 'NONE',  ( 22.18750000000018119, 0.8284271247464157772, 1.999999999999971800 ) ) ;
#5282=VERTEX_POINT ( 'NONE', #20268 ) ;
#5297=CYLINDRICAL_SURFACE ( 'NONE', #576, 2.499999999999999112 ) ;
#5301=CARTESIAN_POINT ( 'NONE',  ( 22.81250000000002132, 0.8284271247461753029, -2.000000000000091926 ) ) ;
#5307=ORIENTED_EDGE ( 'NONE', *, *, #25279, .F. ) ;
#5317=CARTESIAN_POINT ( 'NONE',  ( 18.06250000000005684, -1.097466725451379244, -2.649519052838419153 ) ) ;
#5319=VERTEX_POINT ( 'NONE', #8575 ) ;
#5333=CARTESIAN_POINT ( 'NONE',  ( 23.62500000000000711, -1.414213562372923505, -1.414213562373145550 ) ) ;
#5342=CARTESIAN_POINT ( 'NONE',  ( 17.31250000000010303, -1.097466725451439196, -2.649519052838358757 ) ) ;
#5364=CARTESIAN_POINT ( 'NONE',  ( 15.31250000000006928, -0.8284271247461753029, 1.999999999999911626 ) ) ;
#5369=DIRECTION ( 'NONE',  ( -1.000000000000000000, -1.665334536937731113E-16, 1.526556658859586792E-16 ) ) ;
#5395=VERTEX_POINT ( 'NONE', #13084 ) ;
#5418=CARTESIAN_POINT ( 'NONE',  ( 18.53867513459497829, 1.665334536937734811E-13, 2.499999999999946709 ) ) ;
#5419=CARTESIAN_POINT ( 'NONE',  ( 14.50000000000012434, -1.999999999999779732, -5.551115123125782702E-14 ) ) ;
#5423=ORIENTED_EDGE ( 'NONE', *, *, #9428, .F. ) ;
#5427=CARTESIAN_POINT ( 'NONE',  ( 20.06250000000006750, 2.000000000000151879, 0.8284271247461753029 ) ) ;
#5446=CARTESIAN_POINT ( 'NONE',  ( 14.46132486540527218, 5.551115123125782702E-14, -2.500000000000057732 ) ) ;
#5448=CARTESIAN_POINT ( 'NONE',  ( 24.18750000000015277, 0.8284271247463557142, 2.000000000000031530 ) ) ;
#5451=AXIS2_PLACEMENT_3D ( 'NONE', #16014, #25164, #28230 ) ;
#5453=CARTESIAN_POINT ( 'NONE',  ( -2.081668171172168020E-16, -5.204170427930420051E-17, 2.499999999999999112 ) ) ;
#5463=CARTESIAN_POINT ( 'NONE',  ( 18.62500000000008527, 5.551115123125782702E-14, 2.649519052838333888 ) ) ;
#5483=CARTESIAN_POINT ( 'NONE',  ( 24.93750000000011369, 2.000000000000151879, -0.8284271247462354770 ) ) ;
#5497=CARTESIAN_POINT ( 'NONE',  ( 24.65759742343044536, 1.434127907288146542, -1.856221326699502905 ) ) ;
#5498=EDGE_LOOP ( 'NONE', ( #29944, #24628, #9666, #28397 ) ) ;
#5507=CARTESIAN_POINT ( 'NONE',  ( 19.27382486540524553, -2.499999999999964473, -1.035533905932749299 ) ) ;
#5510=CARTESIAN_POINT ( 'NONE',  ( 16.87500000000000000, 1.414213562373256572, -1.414213562373145550 ) ) ;
#5529=LINE ( 'NONE', #8294, #43 ) ;
#5534=CARTESIAN_POINT ( 'NONE',  ( 10.93750000000009948, 2.000000000000091926, -0.8284271247462354770 ) ) ;
#5574=CARTESIAN_POINT ( 'NONE',  ( 18.31249999999999645, -0.8284271247460553989, 2.000000000000031530 ) ) ;
#5578=ADVANCED_FACE ( 'NONE', ( #27404 ), #8852, .T. ) ;
#5579=CARTESIAN_POINT ( 'NONE',  ( 13.81250000000000000, -2.649519052838178457, 1.097466725451499370 ) ) ;
#5586=DIRECTION ( 'NONE',  ( -8.326672684688674053E-17, -2.081668171172168513E-17, 1.000000000000000000 ) ) ;
#5591=CARTESIAN_POINT ( 'NONE',  ( 19.96132486540530593, 5.551115123125782702E-14, 2.500000000000002220 ) ) ;
#5601=CARTESIAN_POINT ( 'NONE',  ( 22.12500000000006040, 1.414213562373145550, 1.414213562373201061 ) ) ;
#5609=CARTESIAN_POINT ( 'NONE',  ( 24.92558298569622366, 1.541947152209776295, -1.394316296550170531 ) ) ;
#5613=CARTESIAN_POINT ( 'NONE',  ( 17.81250000000009592, -2.649519052838178457, 1.097466725451559322 ) ) ;
#5617=DIRECTION ( 'NONE',  ( -1.000000000000000000, -1.665334536937731113E-16, 1.526556658859586792E-16 ) ) ;
#5624=CARTESIAN_POINT ( 'NONE',  ( 22.72617513459488592, -2.499999999999964473, 1.035533905932749299 ) ) ;
#5632=CARTESIAN_POINT ( 'NONE',  ( 23.50000000000010303, -1.999999999999779732, -5.551115123125782702E-14 ) ) ;
#5641=ORIENTED_EDGE ( 'NONE', *, *, #10974, .T. ) ;
#5642=CARTESIAN_POINT ( 'NONE',  ( 14.37500000000008171, 1.665334536937734811E-13, -2.649519052838444910 ) ) ;
#5655=ORIENTED_EDGE ( 'NONE', *, *, #17078, .F. ) ;
#5661=CARTESIAN_POINT ( 'NONE',  ( 14.75000000000009592, 2.220446049250313081E-13, -2.000000000000057288 ) ) ;
#5665=CARTESIAN_POINT ( 'NONE',  ( 12.08632486540531303, -1.767766952966209892, 1.767766952966431937 ) ) ;
#5682=CARTESIAN_POINT ( 'NONE',  ( 11.37500000000010658, -1.414213562372979016, 1.414213562372979016 ) ) ;
#5693=CARTESIAN_POINT ( 'NONE',  ( 24.93750000000014211, -2.649519052838178457, -1.097466725451619718 ) ) ;
#5695=CARTESIAN_POINT ( 'NONE',  ( 18.72617513459488237, -2.499999999999964473, 1.035533905932689347 ) ) ;
#5725=EDGE_CURVE ( 'NONE', #14931, #17836, #24270, .T. ) ;
#5728=CARTESIAN_POINT ( 'NONE',  ( 17.00000000000015277, 2.000000000000112799, 0.000000000000000000 ) ) ;
#5732=CARTESIAN_POINT ( 'NONE',  ( 14.00000000000006750, -1.873492889144789952, -1.873492889145123019 ) ) ;
#5741=SURFACE_STYLE_USAGE ( .BOTH. , #24481 ) ;
#5750=CARTESIAN_POINT ( 'NONE',  ( 22.37500000000011724, -1.414213562372979016, 1.414213562372979016 ) ) ;
#5752=EDGE_CURVE ( 'NONE', #27492, #24705, #19544, .T. ) ;
#5755=ORIENTED_EDGE ( 'NONE', *, *, #24519, .F. ) ;
#5759=CARTESIAN_POINT ( 'NONE',  ( 24.98686014176553982, 2.013139858234869184, -0.2747217959037423496 ) ) ;
#5765=CARTESIAN_POINT ( 'NONE',  ( 16.43750000000002132, 2.649519052838298805, 1.097466725451559322 ) ) ;
#5768=LINE ( 'NONE', #21638, #9301 ) ;
#5781=CARTESIAN_POINT ( 'NONE',  ( 23.87500000000009237, 1.414213562373256572, -1.414213562373145550 ) ) ;
#5788=CARTESIAN_POINT ( 'NONE',  ( 16.25000000000012434, -1.873492889144845464, -1.873492889145123019 ) ) ;
#5799=CARTESIAN_POINT ( 'NONE',  ( 24.69685486351175996, 1.596793880121103681, -1.664379001782430700 ) ) ;
#5810=CARTESIAN_POINT ( 'NONE',  ( 15.49999999999998579, -1.999999999999835243, 0.000000000000000000 ) ) ;
#5830=CARTESIAN_POINT ( 'NONE',  ( 17.78867513459497829, -2.499999999999835687, -2.220446049250313081E-13 ) ) ;
#5838=CARTESIAN_POINT ( 'NONE',  ( 10.31249999999998934, -0.8284271247461753029, 1.999999999999911626 ) ) ;
#5856=AXIS2_PLACEMENT_3D ( 'NONE', #623, #11898, #28707 ) ;
#5857=EDGE_CURVE ( 'NONE', #26328, #11541, #4184, .T. ) ;
#5860=CARTESIAN_POINT ( 'NONE',  ( 2.081668171172167281E-16, 3.582034040661430693E-16, -2.499999999999999112 ) ) ;
#5880=CARTESIAN_POINT ( 'NONE',  ( 18.00000000000012790, 2.000000000000112799, 0.000000000000000000 ) ) ;
#5902=CIRCLE ( 'NONE', #1507, 6.000000000000000888 ) ;
#5906=CARTESIAN_POINT ( 'NONE',  ( 22.68750000000017764, -0.8284271247460552878, -2.000000000000031530 ) ) ;
#5907=CARTESIAN_POINT ( 'NONE',  ( 19.96132486540530593, 5.551115123125782702E-14, 2.500000000000002220 ) ) ;
#5922=CARTESIAN_POINT ( 'NONE',  ( 2.081668171172167281E-16, 3.582034040661430693E-16, -2.499999999999999112 ) ) ;
#5946=CARTESIAN_POINT ( 'NONE',  ( 11.41367513459493033, 1.767766952966487448, 1.767766952966209892 ) ) ;
#5950=CARTESIAN_POINT ( 'NONE',  ( 15.56250000000000533, 2.649519052838358757, -1.097466725451739622 ) ) ;
#5962=VERTEX_POINT ( 'NONE', #12074 ) ;
#5978=CARTESIAN_POINT ( 'NONE',  ( 16.75000000000015277, 1.665334536937734811E-13, -2.000000000000001776 ) ) ;
#5995=CARTESIAN_POINT ( 'NONE',  ( 16.64882486540528106, 2.500000000000205169, -1.035533905932809473 ) ) ;
#6000=CARTESIAN_POINT ( 'NONE',  ( 11.18750000000003908, 0.8284271247462955401, 2.000000000000031530 ) ) ;
#6009=CARTESIAN_POINT ( 'NONE',  ( 9.500000000000008882, -1.999999999999835243, 0.000000000000000000 ) ) ;
#6031=VERTEX_POINT ( 'NONE', #19263 ) ;
#6035=CARTESIAN_POINT ( 'NONE',  ( 14.31250000000002132, -0.8284271247461152399, 2.000000000000151879 ) ) ;
#6037=AXIS2_PLACEMENT_3D ( 'NONE', #19171, #5007, #2705 ) ;
#6046=VERTEX_POINT ( 'NONE', #10651 ) ;
#6047=CARTESIAN_POINT ( 'NONE',  ( 18.50000000000012790, -1.999999999999835243, 0.000000000000000000 ) ) ;
#6050=CARTESIAN_POINT ( 'NONE',  ( 13.75000000000003908, -1.873492889144900975, 1.873492889144734441 ) ) ;
#6053=EDGE_CURVE ( 'NONE', #16791, #13814, #17419, .T. ) ;
#6054=DIRECTION ( 'NONE',  ( 1.000000000000000000, 1.665334536937735797E-16, 0.000000000000000000 ) ) ;
#6055=DIRECTION ( 'NONE',  ( -1.000000000000000000, -1.665334536937731113E-16, 1.526556658859586792E-16 ) ) ;
#6058=CARTESIAN_POINT ( 'NONE',  ( 24.51662501065472100, 0.2042826450495058288, 2.483374989345329187 ) ) ;
#6084=AXIS2_PLACEMENT_3D ( 'NONE', #23848, #2936, #28430 ) ;
#6085=CARTESIAN_POINT ( 'NONE',  ( 16.50000000000015277, 1.873492889145067508, 1.873492889144734441 ) ) ;
#6098=DIRECTION ( 'NONE',  ( -8.326672684688675286E-17, -2.081668171172168821E-17, 1.000000000000000000 ) ) ;
#6118=ADVANCED_FACE ( 'NONE', ( #1099 ), #3007, .T. ) ;
#6137=CARTESIAN_POINT ( 'NONE',  ( 13.12500000000016342, 1.414213562373145550, 1.414213562373034527 ) ) ;
#6154=CARTESIAN_POINT ( 'NONE',  ( 17.97617513459486105, -1.035533905932568999, -2.499999999999904521 ) ) ;
#6181=CARTESIAN_POINT ( 'NONE',  ( 0.000000000000000000, 0.000000000000000000, 0.000000000000000000 ) ) ;
#6182=FACE_OUTER_BOUND ( 'NONE', #12989, .T. ) ;
#6185=CARTESIAN_POINT ( 'NONE',  ( 16.35117513459494276, 2.500000000000084821, 1.035533905932689347 ) ) ;
#6202=CARTESIAN_POINT ( 'NONE',  ( 14.56249999999998934, -1.999999999999851674, -0.8284271247462354770 ) ) ;
#6205=CARTESIAN_POINT ( 'NONE',  ( 14.62500000000008171, 1.110223024625156540E-13, 2.649519052838333888 ) ) ;
#6214=CARTESIAN_POINT ( 'NONE',  ( 17.83632486540526330, 1.767766952966431937, 1.767766952966376426 ) ) ;
#6254=CARTESIAN_POINT ( 'NONE',  ( 13.41367513459493210, 1.767766952966542959, 1.767766952966376426 ) ) ;
#6259=CARTESIAN_POINT ( 'NONE',  ( 15.18750000000010125, -2.649519052838298805, -1.097466725451559322 ) ) ;
#6285=CARTESIAN_POINT ( 'NONE',  ( 23.33632486540526685, -1.767766952966154381, -1.767766952966542959 ) ) ;
#6299=CARTESIAN_POINT ( 'NONE',  ( 23.87500000000009237, 5.551115123125782702E-14, 2.649519052838333888 ) ) ;
#6304=CARTESIAN_POINT ( 'NONE',  ( 10.97617513459489835, -1.035533905932629173, -2.499999999999904521 ) ) ;
#6315=CARTESIAN_POINT ( 'NONE',  ( 23.81250000000003553, 0.8284271247463557142, -2.000000000000151879 ) ) ;
#6320=CARTESIAN_POINT ( 'NONE',  ( 12.10117513459494276, 1.035533905932929599, -2.499999999999964473 ) ) ;
#6321=CARTESIAN_POINT ( 'NONE',  ( 16.97617513459493566, -1.035533905932568999, -2.499999999999904521 ) ) ;
#6342=CARTESIAN_POINT ( 'NONE',  ( 15.00000000000012434, 2.000000000000112799, 0.000000000000000000 ) ) ;
#6345=CARTESIAN_POINT ( 'NONE',  ( 18.64882486540528106, 2.500000000000084821, -1.035533905932869425 ) ) ;
#6352=CARTESIAN_POINT ( 'NONE',  ( 24.52451905283846401, 1.480436431285038258E-13, 2.475480947161601275 ) ) ;
#6367=CARTESIAN_POINT ( 'NONE',  ( 18.87500000000008527, 1.414213562373256572, -1.414213562373090038 ) ) ;
#6368=VECTOR ( 'NONE', #6445, 1000.000000000000000 ) ;
#6429=CARTESIAN_POINT ( 'NONE',  ( 12.93750000000004086, 2.000000000000151879, -0.8284271247462955401 ) ) ;
#6430=EDGE_CURVE ( 'NONE', #27870, #7693, #18098, .T. ) ;
#6433=CARTESIAN_POINT ( 'NONE',  ( 15.53867513459491967, 1.110223024625156540E-13, 2.499999999999835687 ) ) ;
#6437=CARTESIAN_POINT ( 'NONE',  ( 23.02382486540530948, -1.035533905932629173, 2.499999999999784173 ) ) ;
#6445=DIRECTION ( 'NONE',  ( -1.000000000000000000, -1.665334536937731113E-16, 1.526556658859586792E-16 ) ) ;
#6452=FACE_OUTER_BOUND ( 'NONE', #4240, .T. ) ;
#6457=CARTESIAN_POINT ( 'NONE',  ( 10.66367513459495697, -1.767766952966265404, 1.767766952966376426 ) ) ;
#6462=CARTESIAN_POINT ( 'NONE',  ( 10.00000000000016520, 0.07538101147688137937, 2.429594365314368787 ) ) ;
#6464=VERTEX_POINT ( 'NONE', #13500 ) ;
#6475=CARTESIAN_POINT ( 'NONE',  ( 24.50000000000015987, -1.999999999999835243, -5.551115123125782702E-14 ) ) ;
#6476=DIRECTION ( 'NONE',  ( -8.326672684688675286E-17, -2.081668171172168821E-17, 1.000000000000000000 ) ) ;
#6489=DIRECTION ( 'NONE',  ( 0.000000000000000000, 8.346795477010025210E-14, 1.000000000000000000 ) ) ;
#6505=CARTESIAN_POINT ( 'NONE',  ( 12.37500000000013500, -1.414213562372979016, 1.414213562373034527 ) ) ;
#6514=CARTESIAN_POINT ( 'NONE',  ( 10.00000000000014566, 5.637083940101657433E-14, -6.000000000000056843 ) ) ;
#6527=CARTESIAN_POINT ( 'NONE',  ( 19.37500000000019895, -1.414213562372979016, 1.414213562373034527 ) ) ;
#6529=DIRECTION ( 'NONE',  ( -1.000000000000000000, -1.665334536937731113E-16, 1.526556658859586792E-16 ) ) ;
#6534=CARTESIAN_POINT ( 'NONE',  ( 14.71132486540532902, 2.500000000000057732, -1.665334536937734811E-13 ) ) ;
#6555=( BOUNDED_CURVE ( )  B_SPLINE_CURVE ( 2, ( #21386, #2771, #1327, #5624, #28973, #10741, #7395, #465, #21539 ),
 .UNSPECIFIED., .F., .F. ) 
 B_SPLINE_CURVE_WITH_KNOTS ( ( 3, 2, 2, 2, 3 ),
 ( 0.7968750000000000000, 0.8046875000000000000, 0.8125000000000000000, 0.8203125000000000000, 0.8281250000000000000 ),
 .UNSPECIFIED. ) 
 CURVE ( )  GEOMETRIC_REPRESENTATION_ITEM ( )  RATIONAL_B_SPLINE_CURVE ( ( 1.000000000000000000, 0.9238795325112867385, 1.000000000000000000, 0.9238795325112867385, 1.000000000000000000, 0.9238795325112867385, 1.000000000000000000, 0.9238795325112867385, 1.000000000000000000 ) ) 
 REPRESENTATION_ITEM ( '' )  );
#6563=CARTESIAN_POINT ( 'NONE',  ( 10.56250000000007461, 2.649519052838358757, -1.097466725451559322 ) ) ;
#6580=CARTESIAN_POINT ( 'NONE',  ( 22.50000000000013145, 1.873492889145123019, 1.873492889144845464 ) ) ;
#6600=STYLED_ITEM ( 'NONE', ( #335 ), #2752 ) ;
#6607=CARTESIAN_POINT ( 'NONE',  ( 19.56250000000015632, 2.649519052838419153, -1.097466725451499370 ) ) ;
#6628=CARTESIAN_POINT ( 'NONE',  ( 24.81250000000011724, 0.8284271247463557142, -2.000000000000091926 ) ) ;
#6636=DIRECTION ( 'NONE',  ( -1.000000000000000000, -1.665334536937731113E-16, 1.526556658859586792E-16 ) ) ;
#6652=ORIENTED_EDGE ( 'NONE', *, *, #3065, .F. ) ;
#6656=CARTESIAN_POINT ( 'NONE',  ( 13.18750000000006750, 0.8284271247462955401, 2.000000000000031530 ) ) ;
#6664=CARTESIAN_POINT ( 'NONE',  ( 13.81249999999996980, 0.8284271247461753029, -2.000000000000091926 ) ) ;
#6665=EDGE_LOOP ( 'NONE', ( #28506, #29885 ) ) ;
#6667=CARTESIAN_POINT ( 'NONE',  ( 18.77382486540524908, 2.500000000000144773, 1.035533905932689347 ) ) ;
#6668=ORIENTED_EDGE ( 'NONE', *, *, #6755, .F. ) ;
#6676=AXIS2_PLACEMENT_3D ( 'NONE', #10826, #17895, #8326 ) ;
#6686=CARTESIAN_POINT ( 'NONE',  ( 20.50000000000015632, -1.999999999999890754, -5.551115123125782702E-14 ) ) ;
#6693=SURFACE_STYLE_FILL_AREA ( #18239 ) ;
#6701=( BOUNDED_CURVE ( )  B_SPLINE_CURVE ( 2, ( #15195, #5483, #12756, #26531, #10279, #22096, #14889, #7790, #28829, #24230, #19642, #24527, #10431, #29129, #7948, #3181, #17503, #26818, #5781, #26386, #12455, #12603, #5333, #26672, #5632, #3038, #10129, #3328, #21798, #19499, #23891, #9769, #687, #14265, #232, #9616, #19144, #26178, #19444, #16564, #23461, #2834, #2398, #19296, #7446, #5281, #28618, #10072, #526, #14549, #23603, #25885, #28770, #2978, #14688, #24033, #7740, #2681, #18856, #17148, #7589, #4840, #12106, #11810, #9470, #28329, #9922, #14414, #2542, #12256, #28177, #16857, #21445, #26326, #26471, #12399, #377, #21594, #11965, #5427, #21292, #5126, #19007, #7150, #7306, #16712, #16999, #28481, #21747, #4982, #21147, #26035, #85, #23749, #24627, #10847, #8506, #22504, #17915, #3733, #10225, #8348, #20036, #7888, #6047, #20200, #26619, #5574, #12548, #1278, #971, #13004, #5880, #10372, #22035, #3273, #29550, #15464, #27231, #19727, #15138, #3419, #29383, #24181, #21891, #17755, #15302, #829, #5728, #17447, #8038, #29074, #27079, #26762, #22191, #24789, #3126, #12700, #29222, #12847, #3576, #17602, #26919, #24320, #13168, #22343, #19587, #1439, #14837, #28925, #17301, #10689, #14980, #24468, #8187, #1125, #10523, #19877, #13771, #27682, #6342, #15930, #8974, #2212, #22959, #25082, #25385, #6202, #18366, #30312, #11141, #29694, #25226, #24931, #22653, #20490, #23116, #27527, #8667, #6664, #1594, #20961, #2065, #20341, #11303, #11466, #1897, #20810, #27838, #9121, #4344, #20653, #13460, #10997, #18066, #15776, #30158, #4195, #18516, #18211, #3880, #4039, #6505, #27380, #13313, #6807, #16080, #22803, #23271, #1742, #29848, #16233, #25546, #8827, #4508, #11617, #13612, #30000, #13929, #9272, #18666, #15621, #611, #5056, #21819, #455, #10150, #9845, #28856, #17229, #27759, #24635, #25705, #20495, #18215, #1902, #16084, #4351, #13777, #9740, #28448 ),
 .UNSPECIFIED., .F., .T. ) 
 B_SPLINE_CURVE_WITH_KNOTS ( ( 3, 2, 2, 2, 2, 2, 2, 2, 2, 2, 2, 2, 2, 2, 2, 2, 2, 2, 2, 2, 2, 2, 2, 2, 2, 2, 2, 2, 2, 2, 2, 2, 2, 2, 2, 2, 2, 2, 2, 2, 2, 2, 2, 2, 2, 2, 2, 2, 2, 2, 2, 2, 2, 2, 2, 2, 2, 2, 2, 2, 2, 2, 2, 2, 2, 2, 2, 2, 2, 2, 2, 2, 2, 2, 2, 2, 2, 2, 2, 2, 2, 2, 2, 2, 2, 2, 2, 2, 2, 2, 2, 2, 2, 2, 2, 2, 2, 2, 2, 2, 2, 2, 2, 2, 2, 2, 2, 2, 2, 2, 2, 2, 2, 2, 2, 2, 2, 2, 2, 2, 3 ),
 ( 0.000000000000000000, 0.007812500000000366027, 0.01562500000000073205, 0.02343750000000109981, 0.03125000000000146411, 0.03906250000000183881, 0.04687500000000219963, 0.05468750000000256045, 0.06250000000000292821, 0.07031250000000330291, 0.07812500000000367761, 0.08593750000000402456, 0.09375000000000439926, 0.1015625000000047601, 0.1093750000000051209, 0.1171875000000054956, 0.1250000000000058564, 0.1328125000000062450, 0.1406250000000066058, 0.1484375000000069666, 0.1562500000000073552, 0.1640625000000076883, 0.1718750000000080491, 0.1796875000000084377, 0.1875000000000087985, 0.1953125000000091593, 0.2031250000000095202, 0.2109375000000098810, 0.2187500000000102418, 0.2265625000000106304, 0.2343750000000109912, 0.2421875000000113798, 0.2500000000000117129, 0.2578125000000121014, 0.2656250000000124900, 0.2734375000000128231, 0.2812500000000132117, 0.2890625000000135447, 0.2968750000000139333, 0.3046875000000142664, 0.3125000000000147105, 0.3203125000000150435, 0.3281250000000153766, 0.3359375000000157652, 0.3437500000000160982, 0.3515625000000164868, 0.3593750000000168754, 0.3671875000000172085, 0.3750000000000175970, 0.3828125000000179301, 0.3906250000000183187, 0.3984375000000187073, 0.4062500000000190403, 0.4140625000000194289, 0.4218750000000197620, 0.4296875000000201505, 0.4375000000000204836, 0.4453125000000209277, 0.4531250000000212608, 0.4609375000000215938, 0.4687500000000219824, 0.4765625000000223155, 0.4843750000000227596, 0.4921875000000230926, 0.5000000000000234257, 0.5078125000000237588, 0.5156250000000242029, 0.5234375000000245359, 0.5312500000000249800, 0.5390625000000252021, 0.5468750000000256462, 0.5546875000000260902, 0.5625000000000264233, 0.5703125000000267564, 0.5781250000000270894, 0.5859375000000274225, 0.5937500000000278666, 0.6015625000000281997, 0.6093750000000285327, 0.6171875000000288658, 0.6250000000000294209, 0.6328125000000297540, 0.6406250000000300870, 0.6484375000000304201, 0.6562500000000307532, 0.6640625000000311973, 0.6718750000000315303, 0.6796875000000318634, 0.6875000000000321965, 0.6953125000000325295, 0.7031250000000329736, 0.7109375000000334177, 0.7187500000000337508, 0.7265625000000340838, 0.7343750000000344169, 0.7421875000000348610, 0.7500000000000351941, 0.7578125000000355271, 0.7656250000000358602, 0.7734375000000361933, 0.7812500000000366374, 0.7890625000000369704, 0.7968750000000374145, 0.8046875000000377476, 0.8125000000000380806, 0.8203125000000385247, 0.8281250000000388578, 0.8359375000000391909, 0.8437500000000395239, 0.8515625000000398570, 0.8593750000000403011, 0.8671875000000406342, 0.8750000000000409672, 0.8828125000000414113, 0.8906250000000418554, 0.8984375000000421885, 0.9062500000000425215, 0.9140625000000428546, 0.9218750000000431877, 0.9296875000000436318, 0.9375000000000439648 ),
 .UNSPECIFIED. ) 
 CURVE ( )  GEOMETRIC_REPRESENTATION_ITEM ( )  RATIONAL_B_SPLINE_CURVE ( ( 1.000000000000000000, 0.9238795325112867385, 1.000000000000000000, 0.9238795325112867385, 1.000000000000000000, 0.9238795325112867385, 1.000000000000000000, 0.9238795325112867385, 1.000000000000000000, 0.9238795325112867385, 1.000000000000000000, 0.9238795325112867385, 1.000000000000000000, 0.9238795325112867385, 1.000000000000000000, 0.9238795325112867385, 1.000000000000000000, 0.9238795325112867385, 1.000000000000000000, 0.9238795325112867385, 1.000000000000000000, 0.9238795325112867385, 1.000000000000000000, 0.9238795325112867385, 1.000000000000000000, 0.9238795325112867385, 1.000000000000000000, 0.9238795325112867385, 1.000000000000000000, 0.9238795325112867385, 1.000000000000000000, 0.9238795325112867385, 1.000000000000000000, 0.9238795325112867385, 1.000000000000000000, 0.9238795325112867385, 1.000000000000000000, 0.9238795325112867385, 1.000000000000000000, 0.9238795325112867385, 1.000000000000000000, 0.9238795325112867385, 1.000000000000000000, 0.9238795325112867385, 1.000000000000000000, 0.9238795325112867385, 1.000000000000000000, 0.9238795325112867385, 1.000000000000000000, 0.9238795325112867385, 1.000000000000000000, 0.9238795325112867385, 1.000000000000000000, 0.9238795325112867385, 1.000000000000000000, 0.9238795325112867385, 1.000000000000000000, 0.9238795325112867385, 1.000000000000000000, 0.9238795325112867385, 1.000000000000000000, 0.9238795325112867385, 1.000000000000000000, 0.9238795325112867385, 1.000000000000000000, 0.9238795325112867385, 1.000000000000000000, 0.9238795325112867385, 1.000000000000000000, 0.9238795325112867385, 1.000000000000000000, 0.9238795325112867385, 1.000000000000000000, 0.9238795325112867385, 1.000000000000000000, 0.9238795325112867385, 1.000000000000000000, 0.9238795325112867385, 1.000000000000000000, 0.9238795325112867385, 1.000000000000000000, 0.9238795325112867385, 1.000000000000000000, 0.9238795325112867385, 1.000000000000000000, 0.9238795325112867385, 1.000000000000000000, 0.9238795325112867385, 1.000000000000000000, 0.9238795325112867385, 1.000000000000000000, 0.9238795325112867385, 1.000000000000000000, 0.9238795325112867385, 1.000000000000000000, 0.9238795325112867385, 1.000000000000000000, 0.9238795325112867385, 1.000000000000000000, 0.9238795325112867385, 1.000000000000000000, 0.9238795325112867385, 1.000000000000000000, 0.9238795325112867385, 1.000000000000000000, 0.9238795325112867385, 1.000000000000000000, 0.9238795325112867385, 1.000000000000000000, 0.9238795325112867385, 1.000000000000000000, 0.9238795325112867385, 1.000000000000000000, 0.9238795325112867385, 1.000000000000000000, 0.9238795325112867385, 1.000000000000000000, 0.9238795325112867385, 1.000000000000000000, 0.9238795325112867385, 1.000000000000000000, 0.9238795325112867385, 1.000000000000000000, 0.9238795325112867385, 1.000000000000000000, 0.9238795325112867385, 1.000000000000000000, 0.9238795325112867385, 1.000000000000000000, 0.9238795325112867385, 1.000000000000000000, 0.9238795325112867385, 1.000000000000000000, 0.9238795325112867385, 1.000000000000000000, 0.9238795325112867385, 1.000000000000000000, 0.9238795325112867385, 1.000000000000000000, 0.9238795325112867385, 1.000000000000000000, 0.9238795325112867385, 1.000000000000000000, 0.9238795325112867385, 1.000000000000000000, 0.9238795325112867385, 1.000000000000000000, 0.9238795325112867385, 1.000000000000000000, 0.9238795325112867385, 1.000000000000000000, 0.9238795325112867385, 1.000000000000000000, 0.9238795325112867385, 1.000000000000000000, 0.9238795325112867385, 1.000000000000000000, 0.9238795325112867385, 1.000000000000000000, 0.9238795325112867385, 1.000000000000000000, 0.9238795325112867385, 1.000000000000000000, 0.9238795325112867385, 1.000000000000000000, 0.9238795325112867385, 1.000000000000000000, 0.9238795325112867385, 1.000000000000000000, 0.9238795325112867385, 1.000000000000000000, 0.9238795325112867385, 1.000000000000000000, 0.9238795325112867385, 1.000000000000000000, 0.9238795325112867385, 1.000000000000000000, 0.9238795325112867385, 1.000000000000000000, 0.9238795325112867385, 1.000000000000000000, 0.9238795325112867385, 1.000000000000000000, 0.9238795325112867385, 1.000000000000000000, 0.9238795325112867385, 1.000000000000000000, 0.9238795325112867385, 1.000000000000000000, 0.9238795325112867385, 1.000000000000000000, 0.9238795325112867385, 1.000000000000000000, 0.9238795325112867385, 1.000000000000000000, 0.9238795325112867385, 1.000000000000000000, 0.9238795325112867385, 1.000000000000000000, 0.9238795325112867385, 1.000000000000000000, 0.9238795325112867385, 1.000000000000000000, 0.9238795325112867385, 1.000000000000000000, 0.9238795325112867385, 1.000000000000000000, 0.9238795325112867385, 1.000000000000000000, 0.9238795325112867385, 1.000000000000000000, 0.9238795325112867385, 1.000000000000000000, 0.9238795325112867385, 1.000000000000000000, 0.9238795325112867385, 1.000000000000000000, 0.9238795325112867385, 1.000000000000000000, 0.9238795325112867385, 1.000000000000000000, 0.9238795325112867385, 1.000000000000000000, 0.9238795325112867385, 1.000000000000000000, 0.9238795325112867385, 1.000000000000000000, 0.9238795325112867385, 1.000000000000000000, 0.9238795325112867385, 1.000000000000000000, 0.9238795325112867385, 1.000000000000000000, 0.9238795325112867385, 1.000000000000000000, 0.9238795325112867385, 1.000000000000000000, 0.9238795325112867385, 1.000000000000000000, 0.9238795325108584144, 1.000000000000428324 ) ) 
 REPRESENTATION_ITEM ( '' )  );
#6702=ORIENTED_EDGE ( 'NONE', *, *, #20923, .T. ) ;
#6709=MECHANICAL_DESIGN_GEOMETRIC_PRESENTATION_REPRESENTATION('',(#29240),#14131);
#6717=ADVANCED_FACE ( 'NONE', ( #28890 ), #7856, .T. ) ;
#6723=CARTESIAN_POINT ( 'NONE',  ( 15.72617513459489302, -2.499999999999964473, 1.035533905932869425 ) ) ;
#6734=CARTESIAN_POINT ( 'NONE',  ( 23.31250000000013500, 2.649519052838419153, -1.097466725451619718 ) ) ;
#6745=CARTESIAN_POINT ( 'NONE',  ( 13.00000000000003908, 2.000000000000112799, 0.000000000000000000 ) ) ;
#6749=CARTESIAN_POINT ( 'NONE',  ( 22.96132486540528106, 1.665334536937734811E-13, 2.499999999999946709 ) ) ;
#6755=EDGE_CURVE ( 'NONE', #11541, #13814, #16790, .T. ) ;
#6760=CARTESIAN_POINT ( 'NONE',  ( 21.06250000000011013, -2.649519052838118061, 1.097466725451439196 ) ) ;
#6768=CARTESIAN_POINT ( 'NONE',  ( 17.02382486540524553, -1.035533905932508825, 2.499999999999844569 ) ) ;
#6773=CARTESIAN_POINT ( 'NONE',  ( 20.72617513459479355, -2.499999999999964473, 1.035533905932749299 ) ) ;
#6779=CARTESIAN_POINT ( 'NONE',  ( 15.03867513459491967, 1.665334536937734811E-13, -2.500000000000057732 ) ) ;
#6780=CARTESIAN_POINT ( 'NONE',  ( 23.50000000000010303, -1.999999999999779732, -5.551115123125782702E-14 ) ) ;
#6785=DIRECTION ( 'NONE',  ( -1.000000000000000000, -1.665334536937731113E-16, 1.526556658859586792E-16 ) ) ;
#6799=CARTESIAN_POINT ( 'NONE',  ( 13.43750000000012612, -1.999999999999971800, 0.8284271247462354770 ) ) ;
#6807=CARTESIAN_POINT ( 'NONE',  ( 12.18750000000008349, 0.8284271247463557142, 1.999999999999851674 ) ) ;
#6829=DIRECTION ( 'NONE',  ( -1.000000000000000000, -1.665334536937731113E-16, 1.526556658859586792E-16 ) ) ;
#6841=PRESENTATION_STYLE_ASSIGNMENT (( #9465 ) ) ;
#6843=VERTEX_POINT ( 'NONE', #8627 ) ;
#6867=CARTESIAN_POINT ( 'NONE',  ( 24.50000000000013145, 0.6095397824029125111, -2.424553825690234365 ) ) ;
#6871=CARTESIAN_POINT ( 'NONE',  ( 12.68750000000007638, 2.649519052838538613, 1.097466725451439196 ) ) ;
#6873=CARTESIAN_POINT ( 'NONE',  ( 12.77382486540536455, 2.500000000000084821, 1.035533905932689347 ) ) ;
#6886=CARTESIAN_POINT ( 'NONE',  ( 21.00000000000012790, -1.873492889144789952, -1.873492889145011997 ) ) ;
#6893=CYLINDRICAL_SURFACE ( 'NONE', #25554, 2.499999999999999112 ) ;
#6909=CARTESIAN_POINT ( 'NONE',  ( 20.43750000000011369, 1.097466725451739622, -2.649519052838298805 ) ) ;
#6917=ORIENTED_EDGE ( 'NONE', *, *, #5725, .F. ) ;
#6926=CARTESIAN_POINT ( 'NONE',  ( 10.37500000000007816, 2.649519052838555933, -5.551115123125782702E-14 ) ) ;
#6928=CARTESIAN_POINT ( 'NONE',  ( 23.43750000000010303, -1.999999999999851674, 0.8284271247462955401 ) ) ;
#6957=ORIENTED_EDGE ( 'NONE', *, *, #13213, .T. ) ;
#6972=CARTESIAN_POINT ( 'NONE',  ( 19.47617513459484329, 1.035533905932689347, 2.499999999999964473 ) ) ;
#6986=CARTESIAN_POINT ( 'NONE',  ( 20.00000000000004619, 2.000000000000057288, -5.551115123125782702E-14 ) ) ;
#6987=EDGE_CURVE ( 'NONE', #13194, #15054, #10120, .T. ) ;
#6994=CARTESIAN_POINT ( 'NONE',  ( 10.00000000000012079, -0.6095397824213422133, -2.424553825687569830 ) ) ;
#6996=CARTESIAN_POINT ( 'NONE',  ( 11.96132486540524198, 1.110223024625156540E-13, 2.499999999999835687 ) ) ;
#6999=EDGE_CURVE ( 'NONE', #5282, #24822, #10487, .T. ) ;
#7010=MECHANICAL_DESIGN_GEOMETRIC_PRESENTATION_REPRESENTATION('',(#26143),#14873);
#7023=CARTESIAN_POINT ( 'NONE',  ( 10.50000000000014744, 1.873492889145123019, -1.873492889144956486 ) ) ;
#7028=CARTESIAN_POINT ( 'NONE',  ( 23.85117513459495697, -2.499999999999964473, -1.035533905932869425 ) ) ;
#7043=CARTESIAN_POINT ( 'NONE',  ( 21.93750000000006395, -2.649519052838178457, -1.097466725451439196 ) ) ;
#7063=CARTESIAN_POINT ( 'NONE',  ( 20.12500000000000355, -2.649519052838167354, -1.665334536937734811E-13 ) ) ;
#7070=CARTESIAN_POINT ( 'NONE',  ( 10.00000000000014744, 1.110223024625156540E-13, -5.551115123125782702E-14 ) ) ;
#7082=CARTESIAN_POINT ( 'NONE',  ( 12.81250000000010303, -2.649519052838178457, 1.097466725451499370 ) ) ;
#7083=CARTESIAN_POINT ( 'NONE',  ( 18.96132486540530593, 1.110223024625156540E-13, 2.499999999999724665 ) ) ;
#7084=CARTESIAN_POINT ( 'NONE',  ( 17.81250000000015277, 0.8284271247463557142, -2.000000000000091926 ) ) ;
#7091=CARTESIAN_POINT ( 'NONE',  ( 0.000000000000000000, 0.000000000000000000, 0.000000000000000000 ) ) ;
#7099=EDGE_CURVE ( 'NONE', #4040, #21072, #17043, .T. ) ;
#7101=ORIENTED_EDGE ( 'NONE', *, *, #23170, .T. ) ;
#7114=LINE ( 'NONE', #14660, #16210 ) ;
#7142=ORIENTED_EDGE ( 'NONE', *, *, #20882, .T. ) ;
#7150=CARTESIAN_POINT ( 'NONE',  ( 19.81250000000009237, 0.8284271247463557142, -2.000000000000091926 ) ) ;
#7164=CARTESIAN_POINT ( 'NONE',  ( 23.16367513459499605, 1.767766952966598470, -1.767766952966542959 ) ) ;
#7168=CARTESIAN_POINT ( 'NONE',  ( 21.27382486540515316, -2.499999999999904521, -1.035533905932809473 ) ) ;
#7172=EDGE_CURVE ( 'NONE', #12287, #16041, #18573, .T. ) ;
#7176=CARTESIAN_POINT ( 'NONE',  ( 23.06250000000011013, 2.000000000000151879, 0.8284271247462354770 ) ) ;
#7186=CYLINDRICAL_SURFACE ( 'NONE', #23612, 2.499999999999999112 ) ;
#7192=VERTEX_POINT ( 'NONE', #24515 ) ;
#7194=CARTESIAN_POINT ( 'NONE',  ( 23.87500000000017408, -2.649519052838111843, 0.000000000000000000 ) ) ;
#7200=CARTESIAN_POINT ( 'NONE',  ( -2.081668171172168020E-16, -5.204170427930420051E-17, 2.499999999999999112 ) ) ;
#7216=CARTESIAN_POINT ( 'NONE',  ( 20.31250000000006040, -1.097466725451379244, -2.649519052838419153 ) ) ;
#7230=AXIS2_PLACEMENT_3D ( 'NONE', #9308, #18850, #25736 ) ;
#7237=CARTESIAN_POINT ( 'NONE',  ( 23.96132486540522422, 5.551115123125782702E-14, 2.500000000000002220 ) ) ;
#7248=CARTESIAN_POINT ( 'NONE',  ( 24.82780942950758529, -0.3038553683458247168, -2.156145084836660342 ) ) ;
#7256=FACE_OUTER_BOUND ( 'NONE', #12432, .T. ) ;
#7258=EDGE_LOOP ( 'NONE', ( #21068, #10798, #2570, #19326, #29223 ) ) ;
#7278=EDGE_CURVE ( 'NONE', #5282, #886, #23161, .T. ) ;
#7306=CARTESIAN_POINT ( 'NONE',  ( 19.75000000000009948, 1.665334536937734811E-13, -2.000000000000001776 ) ) ;
#7310=CARTESIAN_POINT ( 'NONE',  ( 15.75000000000006928, -1.873492889144900975, 1.873492889144900975 ) ) ;
#7326=ORIENTED_EDGE ( 'NONE', *, *, #18079, .T. ) ;
#7327=CARTESIAN_POINT ( 'NONE',  ( 22.87500000000000711, 1.414213562373312083, -1.414213562373090038 ) ) ;
#7344=CARTESIAN_POINT ( 'NONE',  ( 17.75000000000015632, -1.873492889144845464, 1.873492889144845464 ) ) ;
#7387=CARTESIAN_POINT ( 'NONE',  ( 12.87500000000016342, -2.649519052838111843, 5.551115123125782702E-14 ) ) ;
#7390=CARTESIAN_POINT ( 'NONE',  ( 17.56250000000009592, -1.999999999999851674, -0.8284271247461753029 ) ) ;
#7395=CARTESIAN_POINT ( 'NONE',  ( 22.91367513459488592, -1.767766952966265404, -1.767766952966598470 ) ) ;
#7418=ORIENTED_EDGE ( 'NONE', *, *, #25279, .T. ) ;
#7446=CARTESIAN_POINT ( 'NONE',  ( 22.25000000000010303, 1.110223024625156540E-13, 1.999999999999946265 ) ) ;
#7448=ORIENTED_EDGE ( 'NONE', *, *, #22570, .T. ) ;
#7454=VECTOR ( 'NONE', #25809, 1000.000000000000000 ) ;
#7465=CARTESIAN_POINT ( 'NONE',  ( 24.10117513459489302, 1.035533905932809473, -2.499999999999904521 ) ) ;
#7467=CARTESIAN_POINT ( 'NONE',  ( 13.71132486540530060, 2.500000000000113243, -1.665334536937734811E-13 ) ) ;
#7469=CARTESIAN_POINT ( 'NONE',  ( 24.50000000000015987, -1.999999999999835243, -5.551115123125782702E-14 ) ) ;
#7482=CARTESIAN_POINT ( 'NONE',  ( 17.68750000000000355, -1.097466725451499370, 2.649519052838298805 ) ) ;
#7504=CARTESIAN_POINT ( 'NONE',  ( 17.37500000000011369, 1.665334536937734811E-13, -2.649519052838444910 ) ) ;
#7509=AXIS2_PLACEMENT_3D ( 'NONE', #28427, #21398, #26133 ) ;
#7515=CARTESIAN_POINT ( 'NONE',  ( 22.16367513459488592, 1.767766952966487448, -1.767766952966598470 ) ) ;
#7523=CARTESIAN_POINT ( 'NONE',  ( 10.93750000000009948, -2.649519052838238409, -1.097466725451439196 ) ) ;
#7526=CARTESIAN_POINT ( 'NONE',  ( 20.50000000000015632, -1.999999999999890754, -5.551115123125782702E-14 ) ) ;
#7540=( BOUNDED_CURVE ( )  B_SPLINE_CURVE ( 2, ( #21387, #19235, #9861, #14499, #12494, #16941, #5665, #7824, #23836 ),
 .UNSPECIFIED., .F., .F. ) 
 B_SPLINE_CURVE_WITH_KNOTS ( ( 3, 2, 2, 2, 3 ),
 ( 0.7656250000000000000, 0.7734375000000000000, 0.7812500000000000000, 0.7890625000000000000, 0.7968750000000000000 ),
 .UNSPECIFIED. ) 
 CURVE ( )  GEOMETRIC_REPRESENTATION_ITEM ( )  RATIONAL_B_SPLINE_CURVE ( ( 1.000000000000000000, 0.9238795325112867385, 1.000000000000000000, 0.9238795325112867385, 1.000000000000000000, 0.9238795325112867385, 1.000000000000000000, 0.9238795325112867385, 1.000000000000000000 ) ) 
 REPRESENTATION_ITEM ( '' )  );
#7548=CARTESIAN_POINT ( 'NONE',  ( 12.43750000000010836, -1.999999999999851674, 0.8284271247462955401 ) ) ;
#7558=UNCERTAINTY_MEASURE_WITH_UNIT (LENGTH_MEASURE( 1.000000000000000082E-05 ), #7899, 'distance_accuracy_value', 'NONE');
#7578=CARTESIAN_POINT ( 'NONE',  ( 17.81250000000015277, 0.8284271247463557142, -2.000000000000091926 ) ) ;
#7589=CARTESIAN_POINT ( 'NONE',  ( 21.25000000000015632, 0.000000000000000000, 2.000000000000057288 ) ) ;
#7598=( NAMED_UNIT ( * ) PLANE_ANGLE_UNIT ( ) SI_UNIT ( $, .RADIAN. ) );
#7603=VECTOR ( 'NONE', #21770, 1000.000000000000000 ) ;
#7613=CARTESIAN_POINT ( 'NONE',  ( 23.18750000000004619, 0.8284271247462955401, 1.999999999999851674 ) ) ;
#7626=CARTESIAN_POINT ( 'NONE',  ( 17.87500000000005684, -2.649519052838167354, -5.551115123125782702E-14 ) ) ;
#7655=CARTESIAN_POINT ( 'NONE',  ( 19.06250000000011013, -2.649519052838238409, 1.097466725451439196 ) ) ;
#7659=CARTESIAN_POINT ( 'NONE',  ( 17.28867513459492145, 2.500000000000113243, -1.110223024625156540E-13 ) ) ;
#7668=( BOUNDED_CURVE ( )  B_SPLINE_CURVE ( 2, ( #15443, #29675, #29983, #3712, #22323, #6185, #8643, #3557, #4020 ),
 .UNSPECIFIED., .F., .T. ) 
 B_SPLINE_CURVE_WITH_KNOTS ( ( 3, 2, 2, 2, 3 ),
 ( 0.3906250000000000000, 0.3984375000000000000, 0.4062500000000000000, 0.4140625000000000000, 0.4218750000000000000 ),
 .UNSPECIFIED. ) 
 CURVE ( )  GEOMETRIC_REPRESENTATION_ITEM ( )  RATIONAL_B_SPLINE_CURVE ( ( 1.000000000000000000, 0.9238795325112867385, 1.000000000000000000, 0.9238795325112867385, 1.000000000000000000, 0.9238795325112867385, 1.000000000000000000, 0.9238795325112867385, 1.000000000000000000 ) ) 
 REPRESENTATION_ITEM ( '' )  );
#7674=EDGE_LOOP ( 'NONE', ( #5307, #23610, #25821, #1469 ) ) ;
#7675=CARTESIAN_POINT ( 'NONE',  ( 19.37500000000019895, -1.414213562372979016, 1.414213562373034527 ) ) ;
#7693=VERTEX_POINT ( 'NONE', #17111 ) ;
#7706=ORIENTED_EDGE ( 'NONE', *, *, #13077, .F. ) ;
#7707=CARTESIAN_POINT ( 'NONE',  ( 10.12500000000007816, 1.414213562373201061, 1.414213562373145550 ) ) ;
#7730=CARTESIAN_POINT ( 'NONE',  ( 17.06250000000001421, 2.000000000000151879, 0.8284271247461753029 ) ) ;
#7740=CARTESIAN_POINT ( 'NONE',  ( 21.50000000000004619, -1.999999999999890754, -1.665334536937734811E-13 ) ) ;
#7742=ORIENTED_EDGE ( 'NONE', *, *, #23552, .T. ) ;
#7758=CARTESIAN_POINT ( 'NONE',  ( 9.562500000000028422, 2.649519052838298805, -1.097466725451559322 ) ) ;
#7771=CARTESIAN_POINT ( 'NONE',  ( 19.12500000000014211, 1.110223024625156540E-13, -2.649519052838444910 ) ) ;
#7772=EDGE_CURVE ( 'NONE', #6031, #27584, #21869, .T. ) ;
#7784=CARTESIAN_POINT ( 'NONE',  ( 24.99999999999999289, 5.550594706083218745E-14, 1.999999999999776179 ) ) ;
#7790=CARTESIAN_POINT ( 'NONE',  ( 24.56250000000017764, -1.999999999999911626, -0.8284271247462354770 ) ) ;
#7794=CARTESIAN_POINT ( 'NONE',  ( 11.10117513459493033, 1.035533905932929599, -2.500000000000024425 ) ) ;
#7795=CARTESIAN_POINT ( 'NONE',  ( 24.50000000000013145, 0.6095397824029125111, -2.424553825690234365 ) ) ;
#7797=CARTESIAN_POINT ( 'NONE',  ( 17.87500000000014211, 1.665334536937734811E-13, 2.649519052838167354 ) ) ;
#7820=CARTESIAN_POINT ( 'NONE',  ( 14.12500000000013678, 1.414213562373201061, 1.414213562373034527 ) ) ;
#7824=CARTESIAN_POINT ( 'NONE',  ( 12.02382486540522599, -1.035533905932629173, 2.499999999999784173 ) ) ;
#7825=SURFACE_STYLE_FILL_AREA ( #26125 ) ;
#7846=( BOUNDED_CURVE ( )  B_SPLINE_CURVE ( 2, ( #21987, #12643, #16694, #4821, #14932, #17398, #920, #15084, #25720 ),
 .UNSPECIFIED., .F., .F. ) 
 B_SPLINE_CURVE_WITH_KNOTS ( ( 3, 2, 2, 2, 3 ),
 ( 0.7031250000000000000, 0.7109375000000000000, 0.7187500000000000000, 0.7265625000000000000, 0.7343750000000000000 ),
 .UNSPECIFIED. ) 
 CURVE ( )  GEOMETRIC_REPRESENTATION_ITEM ( )  RATIONAL_B_SPLINE_CURVE ( ( 1.000000000000000000, 0.9238795325112867385, 1.000000000000000000, 0.9238795325112867385, 1.000000000000000000, 0.9238795325112867385, 1.000000000000000000, 0.9238795325112867385, 1.000000000000000000 ) ) 
 REPRESENTATION_ITEM ( '' )  );
#7856=CYLINDRICAL_SURFACE ( 'NONE', #22907, 2.499999999999999112 ) ;
#7879=CARTESIAN_POINT ( 'NONE',  ( 16.06250000000006040, 2.000000000000151879, 0.8284271247461152399 ) ) ;
#7888=CARTESIAN_POINT ( 'NONE',  ( 18.56250000000004974, -1.999999999999971800, -0.8284271247462354770 ) ) ;
#7899=( LENGTH_UNIT ( ) NAMED_UNIT ( * ) SI_UNIT ( .MILLI., .METRE. ) );
#7916=ORIENTED_EDGE ( 'NONE', *, *, #22991, .T. ) ;
#7923=CIRCLE ( 'NONE', #26586, 5.000000000000000888 ) ;
#7927=CARTESIAN_POINT ( 'NONE',  ( 19.06250000000004619, -1.097466725451379244, -2.649519052838478661 ) ) ;
#7939=( BOUNDED_CURVE ( )  B_SPLINE_CURVE ( 2, ( #26776, #11781, #22814, #9446, #23128, #18679, #11480, #6972, #4359 ),
 .UNSPECIFIED., .F., .T. ) 
 B_SPLINE_CURVE_WITH_KNOTS ( ( 3, 2, 2, 2, 3 ),
 ( 0.5781250000000000000, 0.5859375000000000000, 0.5937500000000000000, 0.6015625000000000000, 0.6093750000000000000 ),
 .UNSPECIFIED. ) 
 CURVE ( )  GEOMETRIC_REPRESENTATION_ITEM ( )  RATIONAL_B_SPLINE_CURVE ( ( 1.000000000000000000, 0.9238795325112867385, 1.000000000000000000, 0.9238795325112867385, 1.000000000000000000, 0.9238795325112867385, 1.000000000000000000, 0.9238795325112867385, 1.000000000000000000 ) ) 
 REPRESENTATION_ITEM ( '' )  );
#7944=CARTESIAN_POINT ( 'NONE',  ( 19.03867513459492500, 1.110223024625156540E-13, -2.500000000000057732 ) ) ;
#7948=CARTESIAN_POINT ( 'NONE',  ( 24.12500000000009237, 1.414213562373201061, 1.414213562373034527 ) ) ;
#7959=CARTESIAN_POINT ( 'NONE',  ( 21.03867513459492500, 1.665334536937734811E-13, -2.500000000000002220 ) ) ;
#7965=ORIENTED_EDGE ( 'NONE', *, *, #9244, .T. ) ;
#7973=CARTESIAN_POINT ( 'NONE',  ( 15.68750000000012612, -0.8284271247459350507, -2.000000000000031530 ) ) ;
#7975=CARTESIAN_POINT ( 'NONE',  ( 24.50000000000010658, 5.545910952697852281E-14, 2.499999999999943601 ) ) ;
#7979=CARTESIAN_POINT ( 'NONE',  ( 13.85117513459488947, -2.499999999999904521, -1.035533905932749299 ) ) ;
#8003=CARTESIAN_POINT ( 'NONE',  ( 10.96132486540515849, 1.110223024625156540E-13, 2.499999999999835687 ) ) ;
#8007=CARTESIAN_POINT ( 'NONE',  ( 25.06250000000014211, -1.097466725451379244, -2.649519052838419153 ) ) ;
#8009=CARTESIAN_POINT ( 'NONE',  ( 18.53867513459497829, 1.665334536937734811E-13, 2.499999999999946709 ) ) ;
#8021=EDGE_CURVE ( 'NONE', #886, #12287, #29285, .T. ) ;
#8031=CARTESIAN_POINT ( 'NONE',  ( 14.25000000000012434, 5.551115123125782702E-14, 2.000000000000001776 ) ) ;
#8038=CARTESIAN_POINT ( 'NONE',  ( 16.87500000000000000, 1.414213562373256572, -1.414213562373145550 ) ) ;
#8042=CARTESIAN_POINT ( 'NONE',  ( 14.75000000000004086, -1.873492889144789952, 1.873492889144845464 ) ) ;
#8045=COLOUR_RGB ( '', 0.09019608, 0.27058824, 0.51372549) ;
#8055=CARTESIAN_POINT ( 'NONE',  ( 18.08632486540531659, -1.767766952966209892, 1.767766952966431937 ) ) ;
#8056=CARTESIAN_POINT ( 'NONE',  ( 21.62500000000017053, -1.414213562372979016, -1.414213562373090038 ) ) ;
#8064=CARTESIAN_POINT ( 'NONE',  ( 24.84150635094622572, -1.291286745249641628E-13, -2.158493649053927044 ) ) ;
#8065=VERTEX_POINT ( 'NONE', #25501 ) ;
#8086=CARTESIAN_POINT ( 'NONE',  ( 0.000000000000000000, 0.000000000000000000, 0.000000000000000000 ) ) ;
#8089=CARTESIAN_POINT ( 'NONE',  ( 2.081668171172167281E-16, 3.582034040661430693E-16, -2.499999999999999112 ) ) ;
#8093=CARTESIAN_POINT ( 'NONE',  ( 16.08632486540520645, -1.767766952966376426, 1.767766952966376426 ) ) ;
#8104=ORIENTED_EDGE ( 'NONE', *, *, #8260, .F. ) ;
#8114=VECTOR ( 'NONE', #24969, 1000.000000000000000 ) ;
#8118=CARTESIAN_POINT ( 'NONE',  ( 13.81249999999996980, 0.8284271247461753029, -2.000000000000091926 ) ) ;
#8136=CARTESIAN_POINT ( 'NONE',  ( 16.58632486540528816, 1.767766952966431937, -1.767766952966487448 ) ) ;
#8139=ORIENTED_EDGE ( 'NONE', *, *, #6755, .T. ) ;
#8149=CARTESIAN_POINT ( 'NONE',  ( 24.87500000000017408, -2.649519052838167354, -5.551115123125782702E-14 ) ) ;
#8160=CARTESIAN_POINT ( 'NONE',  ( -2.081668171172168020E-16, -5.204170427930420051E-17, 2.499999999999999112 ) ) ;
#8165=DIRECTION ( 'NONE',  ( -0.7071067811865455743, -1.644171197757234052E-17, -0.7071067811865495711 ) ) ;
#8187=CARTESIAN_POINT ( 'NONE',  ( 15.37500000000011013, -1.414213562373034527, 1.414213562373034527 ) ) ;
#8205=CARTESIAN_POINT ( 'NONE',  ( 0.000000000000000000, 0.000000000000000000, 0.000000000000000000 ) ) ;
#8211=CARTESIAN_POINT ( 'NONE',  ( 21.68750000000000711, -0.8284271247461753029, -2.000000000000031530 ) ) ;
#8233=CARTESIAN_POINT ( 'NONE',  ( 18.03867513459492145, 1.665334536937734811E-13, -2.500000000000057732 ) ) ;
#8259=CARTESIAN_POINT ( 'NONE',  ( 24.50000000000013145, 0.6095397824029125111, -2.424553825690234365 ) ) ;
#8260=EDGE_CURVE ( 'NONE', #5962, #24536, #25432, .T. ) ;
#8261=ORIENTED_EDGE ( 'NONE', *, *, #28821, .F. ) ;
#8273=CARTESIAN_POINT ( 'NONE',  ( 16.56250000000011369, -1.999999999999911626, -0.8284271247462354770 ) ) ;
#8290=CARTESIAN_POINT ( 'NONE',  ( 24.06250000000009592, -2.649519052838178457, 1.097466725451439196 ) ) ;
#8294=CARTESIAN_POINT ( 'NONE',  ( 2.081668171172167281E-16, 3.582034040661430693E-16, -2.499999999999999112 ) ) ;
#8300=CARTESIAN_POINT ( 'NONE',  ( 10.85117513459490013, -2.499999999999844569, -1.035533905932749299 ) ) ;
#8302=CARTESIAN_POINT ( 'NONE',  ( 19.60117513459486815, -1.035533905932629173, 2.500000000000024425 ) ) ;
#8310=CARTESIAN_POINT ( 'NONE',  ( 24.50000000000015987, 1.873492889145123019, 1.873492889144734441 ) ) ;
#8322=CARTESIAN_POINT ( 'NONE',  ( 24.53656071872807232, -0.3046082907918452598, 2.449202433447952743 ) ) ;
#8326=DIRECTION ( 'NONE',  ( -8.326672684688675286E-17, -2.081668171172168821E-17, 1.000000000000000000 ) ) ;
#8331=FILL_AREA_STYLE ('',( #24611 ) ) ;
#8336=CARTESIAN_POINT ( 'NONE',  ( 15.68750000000012612, -0.8284271247459350507, -2.000000000000031530 ) ) ;
#8348=CARTESIAN_POINT ( 'NONE',  ( 18.68750000000004974, -0.8284271247461753029, -1.999999999999971800 ) ) ;
#8352=CARTESIAN_POINT ( 'NONE',  ( 12.93750000000004086, -2.649519052838298805, -1.097466725451559322 ) ) ;
#8367=EDGE_CURVE ( 'NONE', #23217, #19618, #23397, .T. ) ;
#8418=CARTESIAN_POINT ( 'NONE',  ( 15.50000000000018119, 1.873492889145123019, -1.873492889144956486 ) ) ;
#8424=CIRCLE ( 'NONE', #25598, 6.000000000000001776 ) ;
#8442=CARTESIAN_POINT ( 'NONE',  ( 13.68750000000000178, -0.8284271247459350507, -2.000000000000091926 ) ) ;
#8460=CARTESIAN_POINT ( 'NONE',  ( 12.83632486540528461, 1.767766952966431937, 1.767766952966320915 ) ) ;
#8465=CARTESIAN_POINT ( 'NONE',  ( 10.06250000000005151, 2.000000000000212275, 0.8284271247461152399 ) ) ;
#8486=CARTESIAN_POINT ( 'NONE',  ( 10.47617513459493743, 1.035533905932869425, 2.499999999999844569 ) ) ;
#8492=( BOUNDED_CURVE ( )  B_SPLINE_CURVE ( 2, ( #6867, #18875, #23481 ),
 .UNSPECIFIED., .F., .T. ) 
 B_SPLINE_CURVE_WITH_KNOTS ( ( 3, 3 ),
 ( 0.01315883293259485255, 0.01562500000000000000 ),
 .UNSPECIFIED. ) 
 CURVE ( )  GEOMETRIC_REPRESENTATION_ITEM ( )  RATIONAL_B_SPLINE_CURVE ( ( 0.9671125746063278239, 0.9759710988702530177, 1.000000000000000000 ) ) 
 REPRESENTATION_ITEM ( '' )  );
#8506=CARTESIAN_POINT ( 'NONE',  ( 19.00000000000020961, 2.000000000000223821, -5.551115123125782702E-14 ) ) ;
#8546=CARTESIAN_POINT ( 'NONE',  ( 16.18750000000008527, 1.097466725451559322, -2.649519052838358757 ) ) ;
#8553=ORIENTED_EDGE ( 'NONE', *, *, #22038, .T. ) ;
#8562=CARTESIAN_POINT ( 'NONE',  ( 13.35117513459477401, 2.500000000000084821, 1.035533905932689347 ) ) ;
#8570=CARTESIAN_POINT ( 'NONE',  ( 23.53867513459495342, 1.665334536937734811E-13, 2.499999999999835687 ) ) ;
#8575=CARTESIAN_POINT ( 'NONE',  ( 22.96132486540528106, 1.665334536937734811E-13, 2.499999999999946709 ) ) ;
#8582=ORIENTED_EDGE ( 'NONE', *, *, #6053, .F. ) ;
#8595=CARTESIAN_POINT ( 'NONE',  ( 13.62500000000016520, -1.414213562372923505, -1.414213562373145550 ) ) ;
#8606=CYLINDRICAL_SURFACE ( 'NONE', #20086, 2.499999999999999112 ) ;
#8609=CARTESIAN_POINT ( 'NONE',  ( 23.43750000000004619, 1.097466725451619718, -2.649519052838238409 ) ) ;
#8615=CARTESIAN_POINT ( 'NONE',  ( 5.000000000000087930, 5.551115123125782702E-14, -5.551115123125782702E-14 ) ) ;
#8621=ORIENTED_EDGE ( 'NONE', *, *, #28913, .T. ) ;
#8627=CARTESIAN_POINT ( 'NONE',  ( 23.46132486540525264, 1.110223024625156540E-13, -2.500000000000002220 ) ) ;
#8631=CARTESIAN_POINT ( 'NONE',  ( 24.37500000000014566, -1.414213562373034527, 1.414213562373034527 ) ) ;
#8643=CARTESIAN_POINT ( 'NONE',  ( 16.41367513459479710, 1.767766952966376426, 1.767766952966209892 ) ) ;
#8649=FILL_AREA_STYLE_COLOUR ( '', #2716 ) ;
#8652=( LENGTH_UNIT ( ) NAMED_UNIT ( * ) SI_UNIT ( .MILLI., .METRE. ) );
#8653=ORIENTED_EDGE ( 'NONE', *, *, #7772, .T. ) ;
#8667=CARTESIAN_POINT ( 'NONE',  ( 13.87500000000011013, 1.414213562373312083, -1.414213562373145550 ) ) ;
#8673=CARTESIAN_POINT ( 'NONE',  ( 5.000000000000087041, 5.538625114098749691E-14, 5.999999999999945821 ) ) ;
#8707=CARTESIAN_POINT ( 'NONE',  ( 16.62500000000011369, 1.110223024625156540E-13, 2.649519052838056332 ) ) ;
#8723=CARTESIAN_POINT ( 'NONE',  ( 13.03867513459488947, 5.551115123125782702E-14, -2.500000000000002220 ) ) ;
#8730=CARTESIAN_POINT ( 'NONE',  ( 16.50000000000018119, 1.873492889145067508, -1.873492889144956486 ) ) ;
#8745=EDGE_LOOP ( 'NONE', ( #25780, #3846, #2274, #20528 ) ) ;
#8757=CARTESIAN_POINT ( 'NONE',  ( 11.93750000000008527, 2.000000000000091926, -0.8284271247462354770 ) ) ;
#8794=CARTESIAN_POINT ( 'NONE',  ( 24.31250000000015632, -0.8284271247461152399, 2.000000000000031530 ) ) ;
#8800=CARTESIAN_POINT ( 'NONE',  ( 15.96132486540519047, 1.665334536937734811E-13, 2.500000000000057732 ) ) ;
#8801=CARTESIAN_POINT ( 'NONE',  ( 16.91367513459490723, -1.767766952966209892, -1.767766952966487448 ) ) ;
#8812=FACE_OUTER_BOUND ( 'NONE', #17833, .T. ) ;
#8819=CARTESIAN_POINT ( 'NONE',  ( 12.87500000000008171, 1.414213562373312083, -1.414213562373034527 ) ) ;
#8822=CARTESIAN_POINT ( 'NONE',  ( 21.60117513459502092, -1.035533905932629173, 2.499999999999904521 ) ) ;
#8827=CARTESIAN_POINT ( 'NONE',  ( 11.68750000000000000, -0.8284271247461753029, -1.999999999999971800 ) ) ;
#8830=CARTESIAN_POINT ( 'NONE',  ( 18.22617513459500671, 2.500000000000144773, -1.035533905932869425 ) ) ;
#8838=DIRECTION ( 'NONE',  ( -1.000000000000000000, -1.665334536937731113E-16, 1.526556658859586792E-16 ) ) ;
#8839=CARTESIAN_POINT ( 'NONE',  ( 19.71132486540533435, 2.500000000000224265, -1.110223024625156540E-13 ) ) ;
#8850=CARTESIAN_POINT ( 'NONE',  ( 18.50000000000012790, -1.999999999999835243, 0.000000000000000000 ) ) ;
#8852=CYLINDRICAL_SURFACE ( 'NONE', #15122, 2.499999999999999112 ) ;
#8881=ADVANCED_FACE ( 'NONE', ( #19774 ), #22239, .T. ) ;
#8885=CARTESIAN_POINT ( 'NONE',  ( 11.68750000000009059, 2.649519052838478661, 1.097466725451439196 ) ) ;
#8899=CARTESIAN_POINT ( 'NONE',  ( 21.37500000000011724, 2.649519052838500421, -5.551115123125782702E-14 ) ) ;
#8906=APPLICATION_CONTEXT ( 'automotive_design' ) ;
#8925=CARTESIAN_POINT ( 'NONE',  ( 20.50000000000004619, 1.873492889144956486, -1.873492889144900975 ) ) ;
#8926=CARTESIAN_POINT ( 'NONE',  ( 24.50000000000010658, 5.551115123125782702E-14, -5.551115123125782702E-14 ) ) ;
#8936=CARTESIAN_POINT ( 'NONE',  ( 22.39882486540529172, -1.035533905932568999, -2.499999999999904521 ) ) ;
#8946=CARTESIAN_POINT ( 'NONE',  ( 22.37500000000011724, -1.414213562372979016, 1.414213562372979016 ) ) ;
#8954=CARTESIAN_POINT ( 'NONE',  ( 16.78867513459492145, -2.499999999999891198, -2.775557561562891351E-13 ) ) ;
#8960=FACE_OUTER_BOUND ( 'NONE', #12610, .T. ) ;
#8974=CARTESIAN_POINT ( 'NONE',  ( 14.87500000000011013, 1.414213562373201061, -1.414213562373090038 ) ) ;
#8978=CARTESIAN_POINT ( 'NONE',  ( 18.10117513459491789, 1.035533905932809473, -2.499999999999964473 ) ) ;
#8979=EDGE_CURVE ( 'NONE', #10444, #23217, #20893, .T. ) ;
#8981=DIRECTION ( 'NONE',  ( 1.665334536937731113E-16, -1.000000000000000000, -2.081668171172166973E-17 ) ) ;
#8999=CARTESIAN_POINT ( 'NONE',  ( 21.06250000000004619, 2.000000000000151879, 0.8284271247461152399 ) ) ;
#9006=CARTESIAN_POINT ( 'NONE',  ( 14.89882486540530593, 1.035533905932869425, 2.499999999999904521 ) ) ;
#9012=EDGE_CURVE ( 'NONE', #22842, #1806, #18209, .T. ) ;
#9032=CARTESIAN_POINT ( 'NONE',  ( 11.75000000000009415, 1.873492889145067508, 1.873492889144734441 ) ) ;
#9047=CARTESIAN_POINT ( 'NONE',  ( 22.06250000000009237, -1.097466725451379244, -2.649519052838538613 ) ) ;
#9056=CARTESIAN_POINT ( 'NONE',  ( 13.06249999999998046, 2.000000000000151879, 0.8284271247461152399 ) ) ;
#9058=CARTESIAN_POINT ( 'NONE',  ( -2.081668171172168020E-16, -5.204170427930420051E-17, 2.499999999999999112 ) ) ;
#9069=CARTESIAN_POINT ( 'NONE',  ( 20.25000000000001776, -1.873492889144900975, -1.873492889145178530 ) ) ;
#9082=CARTESIAN_POINT ( 'NONE',  ( 20.66367513459499605, -1.767766952966265404, 1.767766952966320915 ) ) ;
#9088=CARTESIAN_POINT ( 'NONE',  ( 21.62500000000017053, -1.414213562372979016, -1.414213562373090038 ) ) ;
#9097=CARTESIAN_POINT ( 'NONE',  ( 16.66367513459490723, -1.767766952966265404, 1.767766952966376426 ) ) ;
#9116=CARTESIAN_POINT ( 'NONE',  ( 21.85117513459487171, -2.499999999999844569, -1.035533905932809473 ) ) ;
#9121=CARTESIAN_POINT ( 'NONE',  ( 13.18750000000006928, 0.8284271247462955401, 2.000000000000031530 ) ) ;
#9124=CARTESIAN_POINT ( 'NONE',  ( 10.00000000000014566, 1.942114083715059225, -0.8533076016160290322 ) ) ;
#9147=CARTESIAN_POINT ( 'NONE',  ( 20.25000000000015632, 1.110223024625156540E-13, 1.999999999999946265 ) ) ;
#9156=CARTESIAN_POINT ( 'NONE',  ( 11.46132486540535389, 1.110223024625156540E-13, -2.500000000000002220 ) ) ;
#9159=VERTEX_POINT ( 'NONE', #19308 ) ;
#9166=ORIENTED_EDGE ( 'NONE', *, *, #22818, .F. ) ;
#9181=CARTESIAN_POINT ( 'NONE',  ( 10.00000000000017586, -1.873492889144789952, 1.873492889145011997 ) ) ;
#9196=CARTESIAN_POINT ( 'NONE',  ( 21.12500000000011724, 1.665334536937734811E-13, -2.649519052838444910 ) ) ;
#9222=CARTESIAN_POINT ( 'NONE',  ( 20.87500000000008882, 1.110223024625156540E-13, 2.649519052838333888 ) ) ;
#9230=CYLINDRICAL_SURFACE ( 'NONE', #9859, 2.499999999999999112 ) ;
#9236=CARTESIAN_POINT ( 'NONE',  ( 10.75000000000006573, -1.873492889144789952, 1.873492889144845464 ) ) ;
#9238=CARTESIAN_POINT ( 'NONE',  ( 21.87500000000011724, 1.414213562373201061, -1.414213562373090038 ) ) ;
#9242=CARTESIAN_POINT ( 'NONE',  ( 11.78867513459488947, -2.499999999999891198, -2.220446049250313081E-13 ) ) ;
#9243=CARTESIAN_POINT ( 'NONE',  ( 16.03867513459497474, 5.551115123125782702E-14, -2.500000000000057732 ) ) ;
#9244=EDGE_CURVE ( 'NONE', #25491, #6464, #26760, .T. ) ;
#9245=FILL_AREA_STYLE_COLOUR ( '', #12953 ) ;
#9248=CARTESIAN_POINT ( 'NONE',  ( 16.72617513459490723, -2.499999999999904521, 1.035533905932749299 ) ) ;
#9252=CARTESIAN_POINT ( 'NONE',  ( 15.58632486540523132, 1.767766952966487448, -1.767766952966431937 ) ) ;
#9262=AXIS2_PLACEMENT_3D ( 'NONE', #19243, #18955, #26276 ) ;
#9272=CARTESIAN_POINT ( 'NONE',  ( 11.31250000000006573, -0.8284271247460553989, 2.000000000000031530 ) ) ;
#9301=VECTOR ( 'NONE', #5617, 1000.000000000000000 ) ;
#9308=CARTESIAN_POINT ( 'NONE',  ( 9.999999999999980460, 2.500000000000002220, 0.000000000000000000 ) ) ;
#9338=CARTESIAN_POINT ( 'NONE',  ( 11.12500000000016342, -2.649519052838222866, 0.000000000000000000 ) ) ;
#9340=CARTESIAN_POINT ( 'NONE',  ( 12.89882486540518336, 1.035533905932689347, 2.499999999999784173 ) ) ;
#9343=ORIENTED_EDGE ( 'NONE', *, *, #22445, .F. ) ;
#9354=CARTESIAN_POINT ( 'NONE',  ( 24.00000000000013145, -1.873492889144789952, -1.873492889144956486 ) ) ;
#9361=EDGE_CURVE ( 'NONE', #13814, #25453, #7939, .T. ) ;
#9364=CARTESIAN_POINT ( 'NONE',  ( 23.39882486540530593, -1.035533905932689347, -2.500000000000024425 ) ) ;
#9376=CARTESIAN_POINT ( 'NONE',  ( 21.18750000000013500, -2.649519052838178457, -1.097466725451559322 ) ) ;
#9395=CARTESIAN_POINT ( 'NONE',  ( 12.50000000000006750, 1.873492889145011997, 1.873492889144734441 ) ) ;
#9397=CARTESIAN_POINT ( 'NONE',  ( 18.06250000000005684, 2.000000000000151879, 0.8284271247461152399 ) ) ;
#9407=CARTESIAN_POINT ( 'NONE',  ( 24.57479769840429284, -1.155887468185555544, 2.137365870997824491 ) ) ;
#9428=EDGE_CURVE ( 'NONE', #18612, #23931, #8424, .T. ) ;
#9434=B_SPLINE_CURVE_WITH_KNOTS ( 'NONE', 3,
 ( #10856, #29856, #6058, #6352 ),
 .UNSPECIFIED., .F., .F.,
 ( 4, 4 ),
 ( 0.000000000000000000, 0.0006116782145977108518 ),
 .UNSPECIFIED. ) ;
#9446=CARTESIAN_POINT ( 'NONE',  ( 19.22617513459487171, 2.500000000000084821, -1.035533905932929599 ) ) ;
#9458=CARTESIAN_POINT ( 'NONE',  ( 16.75000000000015277, 1.665334536937734811E-13, -2.000000000000001776 ) ) ;
#9463=EDGE_LOOP ( 'NONE', ( #2683, #13497, #18665, #15176 ) ) ;
#9465=SURFACE_STYLE_USAGE ( .BOTH. , #80 ) ;
#9470=CARTESIAN_POINT ( 'NONE',  ( 21.00000000000007461, 2.000000000000057288, 0.000000000000000000 ) ) ;
#9494=CARTESIAN_POINT ( 'NONE',  ( 12.53867513459494631, 1.110223024625156540E-13, 2.500000000000002220 ) ) ;
#9496=CARTESIAN_POINT ( 'NONE',  ( 9.187500000000126121, -2.649519052838178457, -1.097466725451559322 ) ) ;
#9503=CARTESIAN_POINT ( 'NONE',  ( 10.00000000000009237, 2.000000000000112799, 0.000000000000000000 ) ) ;
#9505=EDGE_CURVE ( 'NONE', #25491, #21560, #4051, .T. ) ;
#9513=CARTESIAN_POINT ( 'NONE',  ( 24.12500000000009237, 1.665334536937734811E-13, -2.649519052838333888 ) ) ;
#9514=EDGE_CURVE ( 'NONE', #26264, #7192, #29859, .T. ) ;
#9532=CARTESIAN_POINT ( 'NONE',  ( 20.18750000000012079, -2.649519052838178457, -1.097466725451499370 ) ) ;
#9551=CARTESIAN_POINT ( 'NONE',  ( 10.12500000000002309, 1.110223024625156540E-13, -2.649519052838333888 ) ) ;
#9553=CARTESIAN_POINT ( 'NONE',  ( 19.18750000000004263, 0.8284271247462955401, 2.000000000000031530 ) ) ;
#9570=ORIENTED_EDGE ( 'NONE', *, *, #7172, .T. ) ;
#9573=CARTESIAN_POINT ( 'NONE',  ( 12.37500000000013500, -1.414213562372979016, 1.414213562373034527 ) ) ;
#9606=CARTESIAN_POINT ( 'NONE',  ( 16.50000000000004263, -1.999999999999835243, 0.000000000000000000 ) ) ;
#9616=CARTESIAN_POINT ( 'NONE',  ( 22.81250000000002487, 0.8284271247461753029, -2.000000000000091926 ) ) ;
#9619=CARTESIAN_POINT ( 'NONE',  ( 15.93750000000014921, -2.649519052838238409, -1.097466725451559322 ) ) ;
#9639=CARTESIAN_POINT ( 'NONE',  ( 13.77382486540532014, 2.500000000000084821, 1.035533905932689347 ) ) ;
#9642=CARTESIAN_POINT ( 'NONE',  ( 24.12500000000009237, 1.414213562373201061, 1.414213562373034527 ) ) ;
#9656=ORIENTED_EDGE ( 'NONE', *, *, #9674, .T. ) ;
#9659=CARTESIAN_POINT ( 'NONE',  ( 18.93750000000008171, -2.649519052838238409, -1.097466725451379244 ) ) ;
#9666=ORIENTED_EDGE ( 'NONE', *, *, #22445, .T. ) ;
#9674=EDGE_CURVE ( 'NONE', #6464, #9159, #13715, .T. ) ;
#9683=CARTESIAN_POINT ( 'NONE',  ( 17.25000000000015277, -1.873492889144845464, -1.873492889145123019 ) ) ;
#9688=EDGE_CURVE ( 'NONE', #10444, #28521, #29056, .T. ) ;
#9689=EDGE_CURVE ( 'NONE', #27181, #566, #17402, .T. ) ;
#9704=CARTESIAN_POINT ( 'NONE',  ( 10.43750000000004619, 2.649519052838419153, 1.097466725451559322 ) ) ;
#9711=CARTESIAN_POINT ( 'NONE',  ( 15.16367513459498895, 1.767766952966487448, -1.767766952966431937 ) ) ;
#9720=( BOUNDED_CURVE ( )  B_SPLINE_CURVE ( 2, ( #25357, #25676, #4624, #14056, #11902, #2342, #11742, #21235, #178 ),
 .UNSPECIFIED., .F., .F. ) 
 B_SPLINE_CURVE_WITH_KNOTS ( ( 3, 2, 2, 2, 3 ),
 ( 0.1718750000000000000, 0.1796875000000000000, 0.1875000000000000000, 0.1953125000000000000, 0.2031250000000000000 ),
 .UNSPECIFIED. ) 
 CURVE ( )  GEOMETRIC_REPRESENTATION_ITEM ( )  RATIONAL_B_SPLINE_CURVE ( ( 1.000000000000000000, 0.9238795325112867385, 1.000000000000000000, 0.9238795325112867385, 1.000000000000000000, 0.9238795325112867385, 1.000000000000000000, 0.9238795325112867385, 1.000000000000000000 ) ) 
 REPRESENTATION_ITEM ( '' )  );
#9740=CARTESIAN_POINT ( 'NONE',  ( 10.06249999999967137, 2.000000000003780087, 0.8284271247425472051 ) ) ;
#9757=CARTESIAN_POINT ( 'NONE',  ( 16.87500000000000000, 1.414213562373256572, -1.414213562373145550 ) ) ;
#9765=UNCERTAINTY_MEASURE_WITH_UNIT (LENGTH_MEASURE( 1.000000000000000082E-05 ), #8652, 'distance_accuracy_value', 'NONE');
#9769=CARTESIAN_POINT ( 'NONE',  ( 23.06250000000011013, 2.000000000000151879, 0.8284271247462354770 ) ) ;
#9790=CARTESIAN_POINT ( 'NONE',  ( 24.75000000000010658, 1.665334536937734811E-13, -2.000000000000001776 ) ) ;
#9805=CARTESIAN_POINT ( 'NONE',  ( 17.00000000000001421, -1.873492889144789952, -1.873492889144956486 ) ) ;
#9826=CARTESIAN_POINT ( 'NONE',  ( 16.46132486540524553, 2.220446049250313081E-13, -2.500000000000002220 ) ) ;
#9828=CARTESIAN_POINT ( 'NONE',  ( 18.25000000000012790, -1.873492889144789952, -1.873492889145067508 ) ) ;
#9832=CARTESIAN_POINT ( 'NONE',  ( 18.14882486540516737, -2.499999999999964473, 1.035533905932869425 ) ) ;
#9844=( BOUNDED_CURVE ( )  B_SPLINE_CURVE ( 2, ( #25063, #22785, #22633, #1573, #19098, #11599, #18956, #4786, #23699 ),
 .UNSPECIFIED., .F., .T. ) 
 B_SPLINE_CURVE_WITH_KNOTS ( ( 3, 2, 2, 2, 3 ),
 ( 0.2656250000000000000, 0.2734375000000000000, 0.2812500000000000000, 0.2890625000000000000, 0.2968750000000000000 ),
 .UNSPECIFIED. ) 
 CURVE ( )  GEOMETRIC_REPRESENTATION_ITEM ( )  RATIONAL_B_SPLINE_CURVE ( ( 1.000000000000000000, 0.9238795325112867385, 1.000000000000000000, 0.9238795325112867385, 1.000000000000000000, 0.9238795325112867385, 1.000000000000000000, 0.9238795325112867385, 1.000000000000000000 ) ) 
 REPRESENTATION_ITEM ( '' )  );
#9845=CARTESIAN_POINT ( 'NONE',  ( 10.81250000000001243, 0.8284271247461753029, -2.000000000000091926 ) ) ;
#9849=CARTESIAN_POINT ( 'NONE',  ( 12.06250000000005507, -1.097466725451379244, -2.649519052838419153 ) ) ;
#9853=CARTESIAN_POINT ( 'NONE',  ( 18.56250000000005329, -1.999999999999971800, -0.8284271247462354770 ) ) ;
#9859=AXIS2_PLACEMENT_3D ( 'NONE', #16189, #18622, #10958 ) ;
#9861=CARTESIAN_POINT ( 'NONE',  ( 12.33632486540522954, -1.767766952966320915, -1.767766952966542959 ) ) ;
#9872=SURFACE_STYLE_USAGE ( .BOTH. , #18198 ) ;
#9876=CARTESIAN_POINT ( 'NONE',  ( 12.00000000000012079, 2.000000000000112799, -1.665334536937734811E-13 ) ) ;
#9901=AXIS2_PLACEMENT_3D ( 'NONE', #29974, #29672, #27208 ) ;
#9922=CARTESIAN_POINT ( 'NONE',  ( 20.87500000000014211, 1.414213562373367594, -1.414213562373145550 ) ) ;
#9944=CARTESIAN_POINT ( 'NONE',  ( 23.43750000000010303, -1.999999999999851674, 0.8284271247462955401 ) ) ;
#9957=CARTESIAN_POINT ( 'NONE',  ( 18.00000000000012790, -1.873492889144789952, -1.873492889145123019 ) ) ;
#9982=CARTESIAN_POINT ( 'NONE',  ( 18.06250000000012079, -2.649519052838178457, 1.097466725451499370 ) ) ;
#9990=CARTESIAN_POINT ( 'NONE',  ( 22.52382486540525974, 1.035533905932749299, -2.500000000000024425 ) ) ;
#10005=CARTESIAN_POINT ( 'NONE',  ( 20.62500000000014211, -1.414213562372979016, -1.414213562373145550 ) ) ;
#10024=CARTESIAN_POINT ( 'NONE',  ( 11.06250000000006928, 2.000000000000091926, 0.8284271247461753029 ) ) ;
#10061=CARTESIAN_POINT ( 'NONE',  ( 17.25000000000001421, 1.665334536937734811E-13, 2.000000000000001776 ) ) ;
#10072=CARTESIAN_POINT ( 'NONE',  ( 22.06250000000015632, 2.000000000000212275, 0.8284271247461753029 ) ) ;
#10080=CARTESIAN_POINT ( 'NONE',  ( 0.000000000000000000, 0.000000000000000000, 0.000000000000000000 ) ) ;
#10090=EDGE_CURVE ( 'NONE', #29809, #6843, #12128, .T. ) ;
#10093=EDGE_CURVE ( 'NONE', #30369, #21072, #1298, .T. ) ;
#10110=CARTESIAN_POINT ( 'NONE',  ( 19.81250000000006750, -2.649519052838178457, 1.097466725451499370 ) ) ;
#10120=( BOUNDED_CURVE ( )  B_SPLINE_CURVE ( 2, ( #3230, #10641, #5238, #29037, #930, #14652, #23996, #17108, #8003 ),
 .UNSPECIFIED., .F., .T. ) 
 B_SPLINE_CURVE_WITH_KNOTS ( ( 3, 2, 2, 2, 3 ),
 ( 0.8281250000000000000, 0.8359375000000000000, 0.8437500000000000000, 0.8515625000000000000, 0.8593750000000000000 ),
 .UNSPECIFIED. ) 
 CURVE ( )  GEOMETRIC_REPRESENTATION_ITEM ( )  RATIONAL_B_SPLINE_CURVE ( ( 1.000000000000000000, 0.9238795325112867385, 1.000000000000000000, 0.9238795325112867385, 1.000000000000000000, 0.9238795325112867385, 1.000000000000000000, 0.9238795325112867385, 1.000000000000000000 ) ) 
 REPRESENTATION_ITEM ( '' )  );
#10129=CARTESIAN_POINT ( 'NONE',  ( 23.37500000000000711, -1.414213562373090038, 1.414213562373034527 ) ) ;
#10137=CARTESIAN_POINT ( 'NONE',  ( 17.43750000000009592, 1.097466725451679892, -2.649519052838238409 ) ) ;
#10138=AXIS2_PLACEMENT_3D ( 'NONE', #27665, #10981, #6489 ) ;
#10150=CARTESIAN_POINT ( 'NONE',  ( 10.87499999999996803, 1.414213562373312083, -1.414213562373145550 ) ) ;
#10154=CARTESIAN_POINT ( 'NONE',  ( 17.06250000000001421, 2.000000000000151879, 0.8284271247461753029 ) ) ;
#10157=CARTESIAN_POINT ( 'NONE',  ( 20.53867513459481486, 0.000000000000000000, 2.500000000000002220 ) ) ;
#10177=FACE_OUTER_BOUND ( 'NONE', #26958, .T. ) ;
#10184=CARTESIAN_POINT ( 'NONE',  ( 25.18750000000016698, 1.097466725451679892, -2.649519052838298805 ) ) ;
#10216=CARTESIAN_POINT ( 'NONE',  ( 15.43750000000009770, -1.999999999999851674, 0.8284271247462354770 ) ) ;
#10225=CARTESIAN_POINT ( 'NONE',  ( 18.75000000000015632, 1.110223024625156540E-13, -2.000000000000168310 ) ) ;
#10230=CARTESIAN_POINT ( 'NONE',  ( 15.43750000000009770, 2.649519052838538613, 1.097466725451439196 ) ) ;
#10232=FACE_OUTER_BOUND ( 'NONE', #7674, .T. ) ;
#10236=EDGE_CURVE ( 'NONE', #27584, #5282, #29922, .T. ) ;
#10237=SHAPE_REPRESENTATION_RELATIONSHIP ( 'NONE' , 'NONE' ,  #1893, #1155 ) ;
#10247=CARTESIAN_POINT ( 'NONE',  ( 24.35117513459483263, 2.500000000000144773, 1.035533905932689347 ) ) ;
#10261=CARTESIAN_POINT ( 'NONE',  ( 18.43750000000011724, 2.649519052838478661, 1.097466725451439196 ) ) ;
#10279=CARTESIAN_POINT ( 'NONE',  ( 24.75000000000010658, 1.665334536937734811E-13, -2.000000000000001776 ) ) ;
#10302=CARTESIAN_POINT ( 'NONE',  ( 20.21132486540527751, -2.499999999999835687, -2.220446049250313081E-13 ) ) ;
#10304=CARTESIAN_POINT ( 'NONE',  ( 17.12500000000005684, 1.414213562373090038, 1.414213562373201061 ) ) ;
#10327=CARTESIAN_POINT ( 'NONE',  ( 11.00000000000014921, 2.000000000000112799, 0.000000000000000000 ) ) ;
#10335=ADVANCED_FACE ( 'NONE', ( #26346 ), #19603, .T. ) ;
#10337=CARTESIAN_POINT ( 'NONE',  ( 25.12500000000014566, 1.665334536937734811E-13, -2.649519052838333888 ) ) ;
#10338=ORIENTED_EDGE ( 'NONE', *, *, #18090, .T. ) ;
#10347=CARTESIAN_POINT ( 'NONE',  ( -9.159339953159387393E-16, 5.637083940101630296E-14, -6.000000000000001776 ) ) ;
#10362=CARTESIAN_POINT ( 'NONE',  ( 16.25000000000009948, 1.665334536937734811E-13, 2.000000000000001776 ) ) ;
#10372=CARTESIAN_POINT ( 'NONE',  ( 17.93750000000012434, 2.000000000000091926, -0.8284271247463557142 ) ) ;
#10398=CARTESIAN_POINT ( 'NONE',  ( 21.87500000000011724, 1.414213562373201061, -1.414213562373090038 ) ) ;
#10402=ORIENTED_EDGE ( 'NONE', *, *, #14254, .F. ) ;
#10431=CARTESIAN_POINT ( 'NONE',  ( 24.25000000000018829, 1.110223024625156540E-13, 2.000000000000001776 ) ) ;
#10444=VERTEX_POINT ( 'NONE', #20053 ) ;
#10457=CARTESIAN_POINT ( 'NONE',  ( 14.43750000000014033, -1.999999999999851674, 0.8284271247462955401 ) ) ;
#10477=( BOUNDED_CURVE ( )  B_SPLINE_CURVE ( 2, ( #4569, #9340, #8460, #6873, #20868, #4258, #18274, #23019, #30064 ),
 .UNSPECIFIED., .F., .T. ) 
 B_SPLINE_CURVE_WITH_KNOTS ( ( 3, 2, 2, 2, 3 ),
 ( 0.7343750000000000000, 0.7421875000000000000, 0.7500000000000000000, 0.7578125000000000000, 0.7656250000000000000 ),
 .UNSPECIFIED. ) 
 CURVE ( )  GEOMETRIC_REPRESENTATION_ITEM ( )  RATIONAL_B_SPLINE_CURVE ( ( 1.000000000000000000, 0.9238795325112867385, 1.000000000000000000, 0.9238795325112867385, 1.000000000000000000, 0.9238795325112867385, 1.000000000000000000, 0.9238795325112867385, 1.000000000000000000 ) ) 
 REPRESENTATION_ITEM ( '' )  );
#10480=( GEOMETRIC_REPRESENTATION_CONTEXT ( 3 ) GLOBAL_UNCERTAINTY_ASSIGNED_CONTEXT ( ( #7558 ) ) GLOBAL_UNIT_ASSIGNED_CONTEXT ( ( #7899, #7598, #699 ) ) REPRESENTATION_CONTEXT ( 'NONE', 'WORKASPACE' ) );
#10484=CARTESIAN_POINT ( 'NONE',  ( 10.37500000000005151, -1.414213562373034527, 1.414213562372756972 ) ) ;
#10487=( BOUNDED_CURVE ( )  B_SPLINE_CURVE ( 2, ( #1093, #2939, #24433, #17409, #26435, #28729, #12356, #21706, #644 ),
 .UNSPECIFIED., .F., .T. ) 
 B_SPLINE_CURVE_WITH_KNOTS ( ( 3, 2, 2, 2, 3 ),
 ( 0.2343750000000000000, 0.2421875000000000000, 0.2500000000000000000, 0.2578125000000000000, 0.2656250000000000000 ),
 .UNSPECIFIED. ) 
 CURVE ( )  GEOMETRIC_REPRESENTATION_ITEM ( )  RATIONAL_B_SPLINE_CURVE ( ( 1.000000000000000000, 0.9238795325112867385, 1.000000000000000000, 0.9238795325112867385, 1.000000000000000000, 0.9238795325112867385, 1.000000000000000000, 0.9238795325112867385, 1.000000000000000000 ) ) 
 REPRESENTATION_ITEM ( '' )  );
#10492=CARTESIAN_POINT ( 'NONE',  ( 10.43750000000004619, -1.999999999999851674, 0.8284271247461753029 ) ) ;
#10513=CARTESIAN_POINT ( 'NONE',  ( 16.00000000000007105, 2.000000000000223821, -5.551115123125782702E-14 ) ) ;
#10523=CARTESIAN_POINT ( 'NONE',  ( 15.25000000000012434, 1.110223024625156540E-13, 1.999999999999946265 ) ) ;
#10527=CARTESIAN_POINT ( 'NONE',  ( 13.50000000000006750, 1.873492889145123019, 1.873492889144734441 ) ) ;
#10531=CYLINDRICAL_SURFACE ( 'NONE', #4420, 2.499999999999999112 ) ;
#10532=CARTESIAN_POINT ( 'NONE',  ( 2.081668171172167281E-16, 3.582034040661430693E-16, -2.499999999999999112 ) ) ;
#10551=ORIENTED_EDGE ( 'NONE', *, *, #24519, .T. ) ;
#10556=CARTESIAN_POINT ( 'NONE',  ( 24.90641467890419847, 1.251337131507474831, -1.683925187308909832 ) ) ;
#10560=CARTESIAN_POINT ( 'NONE',  ( 16.31250000000002487, 2.649519052838298805, -1.097466725451499370 ) ) ;
#10562=( BOUNDED_CURVE ( )  B_SPLINE_CURVE ( 2, ( #10746, #1793, #11042, #1171, #17965, #17651, #29434, #17813, #27133 ),
 .UNSPECIFIED., .F., .T. ) 
 B_SPLINE_CURVE_WITH_KNOTS ( ( 3, 2, 2, 2, 3 ),
 ( 0.8906250000000000000, 0.8984375000000000000, 0.9062500000000000000, 0.9140625000000000000, 0.9194088329326726150 ),
 .UNSPECIFIED. ) 
 CURVE ( )  GEOMETRIC_REPRESENTATION_ITEM ( )  RATIONAL_B_SPLINE_CURVE ( ( 1.000000000000000000, 0.9238795325112867385, 1.000000000000000000, 0.9238795325112867385, 1.000000000000000000, 0.9238795325112867385, 1.000000000000000000, 0.9479084336402761046, 0.9671125746068864881 ) ) 
 REPRESENTATION_ITEM ( '' )  );
#10565=CARTESIAN_POINT ( 'NONE',  ( 19.53867513459495342, 5.551115123125782702E-14, 2.500000000000002220 ) ) ;
#10568=CARTESIAN_POINT ( 'NONE',  ( 21.03867513459492500, 1.665334536937734811E-13, -2.500000000000002220 ) ) ;
#10584=CARTESIAN_POINT ( 'NONE',  ( 13.16367513459484861, 1.767766952966431937, -1.767766952966709493 ) ) ;
#10591=CARTESIAN_POINT ( 'NONE',  ( 13.56250000000003375, 2.649519052838358757, -1.097466725451559322 ) ) ;
#10609=ADVANCED_FACE ( 'NONE', ( #2352 ), #29834, .T. ) ;
#10610=EDGE_LOOP ( 'NONE', ( #17795, #24116, #12928, #14031, #19011, #17375, #6652, #8261, #999, #5655, #22792, #23517, #16081, #20654, #10402, #29108, #23157, #24406, #16344, #16661, #13231, #24255, #5755, #12848, #5199, #15856, #18807, #18651, #10959, #24401, #15029, #21190, #3983 ) ) ;
#10611=CARTESIAN_POINT ( 'NONE',  ( 13.93750000000017941, 2.000000000000151879, -0.8284271247462354770 ) ) ;
#10632=CARTESIAN_POINT ( 'NONE',  ( 24.00000000000007816, -1.873492889144789952, 1.873492889144845464 ) ) ;
#10641=CARTESIAN_POINT ( 'NONE',  ( 11.39882486540520468, -1.035533905932568999, -2.499999999999904521 ) ) ;
#10646=CARTESIAN_POINT ( 'NONE',  ( 9.625000000000133227, -1.414213562372979016, -1.414213562373145550 ) ) ;
#10651=CARTESIAN_POINT ( 'NONE',  ( 16.96132486540522066, 1.110223024625156540E-13, 2.500000000000002220 ) ) ;
#10678=CARTESIAN_POINT ( 'NONE',  ( 15.81250000000000178, 0.8284271247462354770, -2.000000000000151879 ) ) ;
#10689=CARTESIAN_POINT ( 'NONE',  ( 15.56250000000003553, -1.999999999999851674, -0.8284271247462354770 ) ) ;
#10703=( NAMED_UNIT ( * ) PLANE_ANGLE_UNIT ( ) SI_UNIT ( $, .RADIAN. ) );
#10707=CARTESIAN_POINT ( 'NONE',  ( 19.83632486540521001, 1.767766952966487448, 1.767766952966320915 ) ) ;
#10708=UNCERTAINTY_MEASURE_WITH_UNIT (LENGTH_MEASURE( 1.000000000000000082E-05 ), #20839, 'distance_accuracy_value', 'NONE');
#10719=CARTESIAN_POINT ( 'NONE',  ( 22.43750000000002842, -1.999999999999851674, 0.8284271247462354770 ) ) ;
#10721=CARTESIAN_POINT ( 'NONE',  ( 10.83632486540525619, 1.767766952966431937, 1.767766952966376426 ) ) ;
#10722=CARTESIAN_POINT ( 'NONE',  ( 13.53867513459486283, 1.110223024625156540E-13, 2.499999999999946709 ) ) ;
#10739=ORIENTED_EDGE ( 'NONE', *, *, #16747, .F. ) ;
#10741=CARTESIAN_POINT ( 'NONE',  ( 22.85117513459491434, -2.499999999999904521, -1.035533905932749299 ) ) ;
#10746=CARTESIAN_POINT ( 'NONE',  ( 10.46132486540518514, 5.551115123125782702E-14, -2.499999999999946709 ) ) ;
#10750=CARTESIAN_POINT ( 'NONE',  ( 13.28867513459505645, 2.500000000000224265, -5.551115123125782702E-14 ) ) ;
#10767=ORIENTED_EDGE ( 'NONE', *, *, #9689, .T. ) ;
#10780=CARTESIAN_POINT ( 'NONE',  ( 16.62500000000013856, -1.414213562372867994, -1.414213562373145550 ) ) ;
#10795=CARTESIAN_POINT ( 'NONE',  ( 17.85117513459488947, -2.499999999999844569, -1.035533905932809473 ) ) ;
#10798=ORIENTED_EDGE ( 'NONE', *, *, #19113, .F. ) ;
#10800=CARTESIAN_POINT ( 'NONE',  ( 10.91367513459493033, -1.767766952966265404, -1.767766952966376426 ) ) ;
#10804=CARTESIAN_POINT ( 'NONE',  ( 19.78867513459489658, -2.499999999999946709, -1.110223024625156540E-13 ) ) ;
#10823=CARTESIAN_POINT ( 'NONE',  ( 24.55536240870550557, -0.7428269089336653197, 2.333994687179698602 ) ) ;
#10826=CARTESIAN_POINT ( 'NONE',  ( 0.000000000000000000, 0.000000000000000000, 0.000000000000000000 ) ) ;
#10828=ORIENTED_EDGE ( 'NONE', *, *, #10938, .T. ) ;
#10836=CARTESIAN_POINT ( 'NONE',  ( 14.56249999999998934, -1.999999999999851674, -0.8284271247462354770 ) ) ;
#10847=CARTESIAN_POINT ( 'NONE',  ( 19.06250000000013500, 2.000000000000091926, 0.8284271247461753029 ) ) ;
#10856=CARTESIAN_POINT ( 'NONE',  ( 24.49999999999999289, 0.6095397824026904665, 2.424553825690067832 ) ) ;
#10860=CARTESIAN_POINT ( 'NONE',  ( 17.58632486540531659, 1.767766952966487448, -1.767766952966598470 ) ) ;
#10889=CARTESIAN_POINT ( 'NONE',  ( 21.47617513459490013, 1.035533905932809473, 2.499999999999844569 ) ) ;
#10903=FACE_OUTER_BOUND ( 'NONE', #22187, .T. ) ;
#10906=CARTESIAN_POINT ( 'NONE',  ( 13.68750000000000178, 2.649519052838298805, 1.097466725451559322 ) ) ;
#10912=VECTOR ( 'NONE', #15940, 1000.000000000000000 ) ;
#10914=PRODUCT ( 'Handle knob', 'Handle knob', '', ( #20211 ) ) ;
#10924=EDGE_LOOP ( 'NONE', ( #13267, #21894, #11524 ) ) ;
#10932=DIRECTION ( 'NONE',  ( -1.000000000000000000, -1.665334536937731113E-16, 1.526556658859586792E-16 ) ) ;
#10935=CARTESIAN_POINT ( 'NONE',  ( 13.66367513459493210, -1.767766952966320915, 1.767766952966431937 ) ) ;
#10938=EDGE_CURVE ( 'NONE', #27584, #12287, #5529, .T. ) ;
#10945=CARTESIAN_POINT ( 'NONE',  ( 23.25000000000018829, -1.873492889144734441, -1.873492889145011997 ) ) ;
#10953=DIRECTION ( 'NONE',  ( 1.526556658859587038E-16, -2.081668171172187002E-17, 1.000000000000000000 ) ) ;
#10957=COLOUR_RGB ( '', 0.66274510, 0.83137255, 0.94901961) ;
#10958=DIRECTION ( 'NONE',  ( -8.326672684688675286E-17, -2.081668171172168821E-17, 1.000000000000000000 ) ) ;
#10959=ORIENTED_EDGE ( 'NONE', *, *, #5246, .F. ) ;
#10966=CARTESIAN_POINT ( 'NONE',  ( 22.12500000000006040, 1.414213562373145550, 1.414213562373201061 ) ) ;
#10972=CARTESIAN_POINT ( 'NONE',  ( 16.46132486540524553, 2.220446049250313081E-13, -2.500000000000002220 ) ) ;
#10974=EDGE_CURVE ( 'NONE', #6046, #29880, #26594, .T. ) ;
#10975=CYLINDRICAL_SURFACE ( 'NONE', #9901, 2.499999999999999112 ) ;
#10981=DIRECTION ( 'NONE',  ( 1.000000000000000000, 1.665334536937731113E-16, -1.526556658859586792E-16 ) ) ;
#10982=ORIENTED_EDGE ( 'NONE', *, *, #9689, .F. ) ;
#10997=CARTESIAN_POINT ( 'NONE',  ( 12.93750000000004263, 2.000000000000151879, -0.8284271247462955401 ) ) ;
#11000=CARTESIAN_POINT ( 'NONE',  ( 15.12500000000008349, 1.665334536937734811E-13, -2.649519052838555933 ) ) ;
#11010=CARTESIAN_POINT ( 'NONE',  ( 17.77382486540514250, 2.500000000000144773, 1.035533905932689347 ) ) ;
#11024=CYLINDRICAL_SURFACE ( 'NONE', #11177, 2.499999999999999112 ) ;
#11025=CARTESIAN_POINT ( 'NONE',  ( 24.85364373589974818, 0.2738724476063931212, -2.146356264100431677 ) ) ;
#11038=DIRECTION ( 'NONE',  ( 0.000000000000000000, 0.000000000000000000, 1.000000000000000000 ) ) ;
#11042=CARTESIAN_POINT ( 'NONE',  ( 10.33632486540525619, -1.767766952966209892, -1.767766952966487448 ) ) ;
#11077=CARTESIAN_POINT ( 'NONE',  ( 12.56250000000007638, -1.999999999999851674, -0.8284271247462354770 ) ) ;
#11081=CARTESIAN_POINT ( 'NONE',  ( 25.00000000000013500, 2.000000000000279332, -5.551115123125782702E-14 ) ) ;
#11091=ORIENTED_EDGE ( 'NONE', *, *, #14651, .T. ) ;
#11098=DIRECTION ( 'NONE',  ( -1.000000000000000000, -1.665334536937731113E-16, 1.526556658859586792E-16 ) ) ;
#11099=CARTESIAN_POINT ( 'NONE',  ( 14.96132486540535567, 5.551115123125782702E-14, 2.500000000000002220 ) ) ;
#11103=CARTESIAN_POINT ( 'NONE',  ( 10.00000000000014744, 1.820239013128537087, 1.173872493019222585 ) ) ;
#11111=CARTESIAN_POINT ( 'NONE',  ( 21.56250000000015987, -1.999999999999911626, -0.8284271247462354770 ) ) ;
#11114=ADVANCED_FACE ( 'NONE', ( #6452 ), #25179, .T. ) ;
#11128=ORIENTED_EDGE ( 'NONE', *, *, #8260, .T. ) ;
#11132=CARTESIAN_POINT ( 'NONE',  ( 12.93750000000004086, 2.000000000000151879, -0.8284271247462955401 ) ) ;
#11141=CARTESIAN_POINT ( 'NONE',  ( 14.37500000000016520, -1.414213562373034527, 1.414213562372979016 ) ) ;
#11142=ORIENTED_EDGE ( 'NONE', *, *, #22400, .T. ) ;
#11145=CARTESIAN_POINT ( 'NONE',  ( 10.00000000000014566, -0.2706188729083223721, -2.470526507789089443 ) ) ;
#11154=DIRECTION ( 'NONE',  ( -1.000000000000000000, -1.665334536937731113E-16, 1.526556658859586792E-16 ) ) ;
#11169=CARTESIAN_POINT ( 'NONE',  ( 18.75000000000015632, 1.110223024625156540E-13, -2.000000000000168310 ) ) ;
#11176=CARTESIAN_POINT ( 'NONE',  ( 14.58632486540512119, 1.767766952966542959, -1.767766952966487448 ) ) ;
#11177=AXIS2_PLACEMENT_3D ( 'NONE', #1310, #3448, #29103 ) ;
#11194=ORIENTED_EDGE ( 'NONE', *, *, #17850, .T. ) ;
#11211=( BOUNDED_CURVE ( )  B_SPLINE_CURVE ( 2, ( #16265, #9006, #30344, #1773, #6534, #15957, #11176, #28325, #17144 ),
 .UNSPECIFIED., .F., .T. ) 
 B_SPLINE_CURVE_WITH_KNOTS ( ( 3, 2, 2, 2, 3 ),
 ( 0.6093750000000000000, 0.6171875000000000000, 0.6250000000000000000, 0.6328125000000000000, 0.6406250000000000000 ),
 .UNSPECIFIED. ) 
 CURVE ( )  GEOMETRIC_REPRESENTATION_ITEM ( )  RATIONAL_B_SPLINE_CURVE ( ( 1.000000000000000000, 0.9238795325112867385, 1.000000000000000000, 0.9238795325112867385, 1.000000000000000000, 0.9238795325112867385, 1.000000000000000000, 0.9238795325112867385, 1.000000000000000000 ) ) 
 REPRESENTATION_ITEM ( '' )  );
#11217=ORIENTED_EDGE ( 'NONE', *, *, #7172, .F. ) ;
#11223=EDGE_CURVE ( 'NONE', #24705, #25491, #15717, .T. ) ;
#11232=CARTESIAN_POINT ( 'NONE',  ( 13.50000000000015099, -1.999999999999890754, -5.551115123125782702E-14 ) ) ;
#11248=CARTESIAN_POINT ( 'NONE',  ( 20.75000000000012790, 1.873492889145011997, 1.873492889144845464 ) ) ;
#11260=CARTESIAN_POINT ( 'NONE',  ( 10.00000000000014744, 1.738740874279711246, 1.328116326731191510 ) ) ;
#11263=CARTESIAN_POINT ( 'NONE',  ( 21.46132486540527751, 5.551115123125782702E-14, -2.500000000000002220 ) ) ;
#11268=CARTESIAN_POINT ( 'NONE',  ( 23.31250000000007461, -0.8284271247460552878, 2.000000000000091926 ) ) ;
#11269=CYLINDRICAL_SURFACE ( 'NONE', #27440, 2.499999999999999112 ) ;
#11277=CARTESIAN_POINT ( 'NONE',  ( 12.53867513459494631, 1.110223024625156540E-13, 2.500000000000002220 ) ) ;
#11294=CARTESIAN_POINT ( 'NONE',  ( 13.50000000000015099, -1.999999999999890754, -5.551115123125782702E-14 ) ) ;
#11303=CARTESIAN_POINT ( 'NONE',  ( 13.50000000000015099, -1.999999999999890754, -5.551115123125782702E-14 ) ) ;
#11330=CARTESIAN_POINT ( 'NONE',  ( 19.43750000000013145, -1.999999999999851674, 0.8284271247462354770 ) ) ;
#11360=( BOUNDED_CURVE ( )  B_SPLINE_CURVE ( 2, ( #5591, #14995, #10707, #3748, #8839, #24645, #24800, #20356, #29396 ),
 .UNSPECIFIED., .F., .F. ) 
 B_SPLINE_CURVE_WITH_KNOTS ( ( 3, 2, 2, 2, 3 ),
 ( 0.2968750000000000000, 0.3046875000000000000, 0.3125000000000000000, 0.3203125000000000000, 0.3281250000000000000 ),
 .UNSPECIFIED. ) 
 CURVE ( )  GEOMETRIC_REPRESENTATION_ITEM ( )  RATIONAL_B_SPLINE_CURVE ( ( 1.000000000000000000, 0.9238795325112867385, 1.000000000000000000, 0.9238795325112867385, 1.000000000000000000, 0.9238795325112867385, 1.000000000000000000, 0.9238795325112867385, 1.000000000000000000 ) ) 
 REPRESENTATION_ITEM ( '' )  );
#11385=CARTESIAN_POINT ( 'NONE',  ( 23.93750000000015277, -2.649519052838178457, -1.097466725451559322 ) ) ;
#11393=CARTESIAN_POINT ( 'NONE',  ( 13.18750000000006750, 0.8284271247462955401, 2.000000000000031530 ) ) ;
#11411=CARTESIAN_POINT ( 'NONE',  ( 22.56250000000008527, 2.649519052838478661, -1.097466725451499370 ) ) ;
#11423=DIRECTION ( 'NONE',  ( -8.326672684688675286E-17, -2.081668171172168821E-17, 1.000000000000000000 ) ) ;
#11426=CARTESIAN_POINT ( 'NONE',  ( 21.96132486540530593, 1.665334536937734811E-13, 2.499999999999946709 ) ) ;
#11431=CARTESIAN_POINT ( 'NONE',  ( 18.97617513459490723, -1.035533905932568999, -2.499999999999964473 ) ) ;
#11433=CARTESIAN_POINT ( 'NONE',  ( 23.93750000000006750, 2.000000000000151879, -0.8284271247462955401 ) ) ;
#11440=CARTESIAN_POINT ( 'NONE',  ( -2.081668171172168020E-16, -5.204170427930420051E-17, 2.499999999999999112 ) ) ;
#11466=CARTESIAN_POINT ( 'NONE',  ( 13.43750000000012434, -1.999999999999971800, 0.8284271247462354770 ) ) ;
#11480=CARTESIAN_POINT ( 'NONE',  ( 19.41367513459493921, 1.767766952966487448, 1.767766952966098870 ) ) ;
#11524=ORIENTED_EDGE ( 'NONE', *, *, #2956, .T. ) ;
#11525=CARTESIAN_POINT ( 'NONE',  ( 10.31250000000007994, -1.097466725451499370, -2.649519052838358757 ) ) ;
#11539=CARTESIAN_POINT ( 'NONE',  ( 21.25000000000013145, 1.873492889145067508, -1.873492889145067508 ) ) ;
#11541=VERTEX_POINT ( 'NONE', #5418 ) ;
#11548=CARTESIAN_POINT ( 'NONE',  ( 11.50000000000006573, -1.999999999999835243, 0.000000000000000000 ) ) ;
#11551=ADVANCED_FACE ( 'NONE', ( #14830 ), #23878, .T. ) ;
#11572=CARTESIAN_POINT ( 'NONE',  ( 20.03867513459486815, 1.665334536937734811E-13, -2.500000000000057732 ) ) ;
#11580=CARTESIAN_POINT ( 'NONE',  ( 18.85117513459493566, -2.499999999999904521, -1.035533905932689347 ) ) ;
#11581=DIRECTION ( 'NONE',  ( -1.000000000000000000, -1.665334536937731113E-16, 1.526556658859586792E-16 ) ) ;
#11582=CARTESIAN_POINT ( 'NONE',  ( 22.68750000000017764, -0.8284271247460552878, -2.000000000000031530 ) ) ;
#11595=CARTESIAN_POINT ( 'NONE',  ( 10.00000000000014744, 1.108974023722453239E-13, 5.999999999999945821 ) ) ;
#11599=CARTESIAN_POINT ( 'NONE',  ( 14.35117513459479177, 2.500000000000024425, 1.035533905932689347 ) ) ;
#11617=CARTESIAN_POINT ( 'NONE',  ( 11.56250000000009237, -1.999999999999851674, -0.8284271247462354770 ) ) ;
#11618=EDGE_LOOP ( 'NONE', ( #21552, #7742, #10767, #9343 ) ) ;
#11620=CARTESIAN_POINT ( 'NONE',  ( 18.71132486540527751, 2.500000000000168754, -5.551115123125782702E-14 ) ) ;
#11644=CARTESIAN_POINT ( 'NONE',  ( 18.93750000000016698, 2.000000000000091926, -0.8284271247462354770 ) ) ;
#11678=ORIENTED_EDGE ( 'NONE', *, *, #29309, .T. ) ;
#11679=CARTESIAN_POINT ( 'NONE',  ( 12.37500000000007994, 1.665334536937734811E-13, -2.649519052838500421 ) ) ;
#11681=CARTESIAN_POINT ( 'NONE',  ( 15.60117513459495342, -1.035533905932689347, 2.499999999999904521 ) ) ;
#11696=CARTESIAN_POINT ( 'NONE',  ( 20.56250000000008171, 1.097466725451679892, 2.649519052838298805 ) ) ;
#11715=CARTESIAN_POINT ( 'NONE',  ( 23.06250000000002487, -2.649519052838298805, 1.097466725451499370 ) ) ;
#11718=DIRECTION ( 'NONE',  ( 0.000000000000000000, -2.081668171172248016E-17, 1.000000000000000000 ) ) ;
#11734=CARTESIAN_POINT ( 'NONE',  ( 14.53867513459486460, 1.665334536937734811E-13, 2.499999999999835687 ) ) ;
#11735=CARTESIAN_POINT ( 'NONE',  ( 18.75000000000015632, 1.110223024625156540E-13, -2.000000000000168310 ) ) ;
#11741=CARTESIAN_POINT ( 'NONE',  ( 11.53867513459497296, 5.551115123125782702E-14, 2.500000000000002220 ) ) ;
#11742=CARTESIAN_POINT ( 'NONE',  ( 12.91367513459493210, -1.767766952966209892, -1.767766952966487448 ) ) ;
#11753=DIRECTION ( 'NONE',  ( -8.326672684688675286E-17, -2.081668171172168821E-17, 1.000000000000000000 ) ) ;
#11768=EDGE_LOOP ( 'NONE', ( #24067, #18772, #11128, #25305 ) ) ;
#11781=CARTESIAN_POINT ( 'NONE',  ( 19.10117513459493566, 1.035533905932809473, -2.499999999999964473 ) ) ;
#11808=ORIENTED_EDGE ( 'NONE', *, *, #3430, .T. ) ;
#11810=CARTESIAN_POINT ( 'NONE',  ( 21.06250000000004619, 2.000000000000151879, 0.8284271247461153509 ) ) ;
#11831=EDGE_CURVE ( 'NONE', #26790, #23931, #7923, .T. ) ;
#11836=CARTESIAN_POINT ( 'NONE',  ( 9.812500000000087041, 1.097466725451679892, 2.649519052838298805 ) ) ;
#11838=CARTESIAN_POINT ( 'NONE',  ( 15.78867513459494809, -2.499999999999946709, -2.220446049250313081E-13 ) ) ;
#11842=CARTESIAN_POINT ( 'NONE',  ( 9.750000000000119016, 1.665334536937734811E-13, -1.999999999999890754 ) ) ;
#11850=CARTESIAN_POINT ( 'NONE',  ( 22.43750000000008882, 2.649519052838419153, 1.097466725451499370 ) ) ;
#11873=CYLINDRICAL_SURFACE ( 'NONE', #24311, 2.499999999999999112 ) ;
#11875=CARTESIAN_POINT ( 'NONE',  ( 21.37500000000019895, 1.110223024625156540E-13, -2.649519052838333888 ) ) ;
#11881=ORIENTED_EDGE ( 'NONE', *, *, #28809, .F. ) ;
#11882=DIRECTION ( 'NONE',  ( -1.000000000000000000, -1.665334536937731113E-16, 1.526556658859586792E-16 ) ) ;
#11887=VERTEX_POINT ( 'NONE', #6433 ) ;
#11890=CIRCLE ( 'NONE', #24088, 6.000000000000001776 ) ;
#11892=CARTESIAN_POINT ( 'NONE',  ( 10.03867513459497118, 1.110223024625156540E-13, -2.500000000000113243 ) ) ;
#11893=CARTESIAN_POINT ( 'NONE',  ( 11.31250000000006395, 2.649519052838419153, -1.097466725451559322 ) ) ;
#11895=CARTESIAN_POINT ( 'NONE',  ( 20.18750000000014566, 0.8284271247463557142, 1.999999999999911626 ) ) ;
#11898=DIRECTION ( 'NONE',  ( -1.000000000000000000, -1.665334536937731113E-16, 1.526556658859586792E-16 ) ) ;
#11902=CARTESIAN_POINT ( 'NONE',  ( 12.78867513459486283, -2.499999999999891198, -2.220446049250313081E-13 ) ) ;
#11903=PRESENTATION_STYLE_ASSIGNMENT (( #23980 ) ) ;
#11904=CARTESIAN_POINT ( 'NONE',  ( 24.78514766611641562, -1.168806754308282292, -1.887491515121927588 ) ) ;
#11935=CARTESIAN_POINT ( 'NONE',  ( 10.53867513459491612, 5.551115123125782702E-14, 2.499999999999724665 ) ) ;
#11955=CARTESIAN_POINT ( 'NONE',  ( 16.56250000000011369, -1.999999999999911626, -0.8284271247462354770 ) ) ;
#11965=CARTESIAN_POINT ( 'NONE',  ( 20.12500000000011369, 1.414213562373201061, 1.414213562373034527 ) ) ;
#11970=CARTESIAN_POINT ( 'NONE',  ( 15.81250000000006395, -2.649519052838178457, 1.097466725451439196 ) ) ;
#11987=CARTESIAN_POINT ( 'NONE',  ( 24.62500000000012079, -1.414213562372923505, -1.414213562373145550 ) ) ;
#12001=CARTESIAN_POINT ( 'NONE',  ( 20.00000000000018474, -1.873492889144845464, -1.873492889144956486 ) ) ;
#12020=CARTESIAN_POINT ( 'NONE',  ( 18.37500000000002842, 1.665334536937734811E-13, -2.649519052838444910 ) ) ;
#12025=CARTESIAN_POINT ( 'NONE',  ( 2.081668171172167281E-16, 3.582034040661430693E-16, -2.499999999999999112 ) ) ;
#12027=CARTESIAN_POINT ( 'NONE',  ( 22.08632486540518158, -1.767766952966320915, 1.767766952966320915 ) ) ;
#12030=ORIENTED_EDGE ( 'NONE', *, *, #10090, .T. ) ;
#12040=CARTESIAN_POINT ( 'NONE',  ( 11.18750000000003908, 1.097466725451679892, -2.649519052838298805 ) ) ;
#12042=MECHANICAL_DESIGN_GEOMETRIC_PRESENTATION_REPRESENTATION('',(#6600),#5131);
#12043=CARTESIAN_POINT ( 'NONE',  ( 17.87500000000008527, 1.414213562373312083, -1.414213562373145550 ) ) ;
#12051=CARTESIAN_POINT ( 'NONE',  ( 15.89882486540525974, 1.035533905932869425, 2.499999999999844569 ) ) ;
#12056=( LENGTH_UNIT ( ) NAMED_UNIT ( * ) SI_UNIT ( .MILLI., .METRE. ) );
#12060=CARTESIAN_POINT ( 'NONE',  ( 12.18750000000008349, 0.8284271247463557142, 1.999999999999851674 ) ) ;
#12074=CARTESIAN_POINT ( 'NONE',  ( 22.03867513459498184, 1.110223024625156540E-13, -2.500000000000057732 ) ) ;
#12094=EDGE_CURVE ( 'NONE', #24705, #26328, #21216, .T. ) ;
#12106=CARTESIAN_POINT ( 'NONE',  ( 21.12500000000011724, 1.414213562373201061, 1.414213562373034527 ) ) ;
#12128=( BOUNDED_CURVE ( )  B_SPLINE_CURVE ( 2, ( #15831, #1338, #15516, #27577, #3932, #13361, #22855, #20254, #24529 ),
 .UNSPECIFIED., .F., .T. ) 
 B_SPLINE_CURVE_WITH_KNOTS ( ( 3, 2, 2, 2, 3 ),
 ( 0.04687500000000000000, 0.05468750000000000000, 0.06250000000000000000, 0.07031250000000000000, 0.07812500000000000000 ),
 .UNSPECIFIED. ) 
 CURVE ( )  GEOMETRIC_REPRESENTATION_ITEM ( )  RATIONAL_B_SPLINE_CURVE ( ( 1.000000000000000000, 0.9238795325112867385, 1.000000000000000000, 0.9238795325112867385, 1.000000000000000000, 0.9238795325112867385, 1.000000000000000000, 0.9238795325112867385, 1.000000000000000000 ) ) 
 REPRESENTATION_ITEM ( '' )  );
#12135=CARTESIAN_POINT ( 'NONE',  ( 20.53867513459481486, 0.000000000000000000, 2.500000000000002220 ) ) ;
#12145=CARTESIAN_POINT ( 'NONE',  ( 17.25000000000012790, 1.873492889145123019, -1.873492889144956486 ) ) ;
#12168=CARTESIAN_POINT ( 'NONE',  ( 17.12500000000011369, -2.649519052838111843, 0.000000000000000000 ) ) ;
#12183=CARTESIAN_POINT ( 'NONE',  ( 22.03867513459498184, 1.110223024625156540E-13, -2.500000000000057732 ) ) ;
#12191=CARTESIAN_POINT ( 'NONE',  ( 11.93750000000008527, -2.649519052838178457, -1.097466725451559322 ) ) ;
#12192=CARTESIAN_POINT ( 'NONE',  ( 19.02382486540536632, -1.035533905932689347, 2.499999999999904521 ) ) ;
#12200=CARTESIAN_POINT ( 'NONE',  ( 15.10117513459490013, 1.035533905932809473, -2.499999999999904521 ) ) ;
#12201=CARTESIAN_POINT ( 'NONE',  ( 24.69040286737535794, -2.307700622106291455, -0.1780978345574568689 ) ) ;
#12205=CARTESIAN_POINT ( 'NONE',  ( 15.52382486540526507, 1.035533905932809473, -2.499999999999904521 ) ) ;
#12209=( NAMED_UNIT ( * ) PLANE_ANGLE_UNIT ( ) SI_UNIT ( $, .RADIAN. ) );
#12215=CARTESIAN_POINT ( 'NONE',  ( 11.87500000000007994, 1.414213562373312083, -1.414213562373090038 ) ) ;
#12256=CARTESIAN_POINT ( 'NONE',  ( 20.68750000000011369, -0.8284271247459952248, -1.999999999999971800 ) ) ;
#12282=CARTESIAN_POINT ( 'NONE',  ( 20.47617513459485394, 1.035533905932869425, 2.499999999999904521 ) ) ;
#12287=VERTEX_POINT ( 'NONE', #7959 ) ;
#12291=CARTESIAN_POINT ( 'NONE',  ( 18.37500000000011369, 2.649519052838444910, -1.110223024625156540E-13 ) ) ;
#12324=CARTESIAN_POINT ( 'NONE',  ( 22.77382486540519224, 2.500000000000144773, 1.035533905932689347 ) ) ;
#12329=ORIENTED_EDGE ( 'NONE', *, *, #23170, .F. ) ;
#12351=VERTEX_POINT ( 'NONE', #13682 ) ;
#12355=CIRCLE ( 'NONE', #26532, 5.000000000000001776 ) ;
#12356=CARTESIAN_POINT ( 'NONE',  ( 20.58632486540526330, 1.767766952966487448, -1.767766952966376426 ) ) ;
#12359=VECTOR ( 'NONE', #881, 1000.000000000000000 ) ;
#12399=CARTESIAN_POINT ( 'NONE',  ( 20.31250000000011724, -0.8284271247461153509, 2.000000000000031530 ) ) ;
#12404=CARTESIAN_POINT ( 'NONE',  ( 15.68750000000015277, -1.097466725451499370, 2.649519052838118061 ) ) ;
#12407=DIRECTION ( 'NONE',  ( -1.000000000000000000, -1.665334536937731113E-16, 1.526556658859586792E-16 ) ) ;
#12423=CARTESIAN_POINT ( 'NONE',  ( 9.687499999999998224, 2.649519052838419153, 1.097466725451499370 ) ) ;
#12425=FACE_OUTER_BOUND ( 'NONE', #7258, .T. ) ;
#12426=LINE ( 'NONE', #5453, #7603 ) ;
#12432=EDGE_LOOP ( 'NONE', ( #10551, #15536, #15918, #27667 ) ) ;
#12435=CARTESIAN_POINT ( 'NONE',  ( 17.93750000000006395, -2.649519052838178457, -1.097466725451559322 ) ) ;
#12455=CARTESIAN_POINT ( 'NONE',  ( 23.75000000000013145, 1.665334536937734811E-13, -2.000000000000057288 ) ) ;
#12463=CARTESIAN_POINT ( 'NONE',  ( 18.18750000000000000, -2.649519052838298805, -1.097466725451559322 ) ) ;
#12471=CARTESIAN_POINT ( 'NONE',  ( 17.03867513459494987, 1.665334536937734811E-13, -2.500000000000002220 ) ) ;
#12475=CARTESIAN_POINT ( 'NONE',  ( 25.00000000000013500, 2.000000000000279332, -5.551115123125782702E-14 ) ) ;
#12489=CARTESIAN_POINT ( 'NONE',  ( 14.93750000000010303, 2.000000000000151879, -0.8284271247462955401 ) ) ;
#12494=CARTESIAN_POINT ( 'NONE',  ( 12.21132486540527040, -2.499999999999946709, -2.220446049250313081E-13 ) ) ;
#12539=CARTESIAN_POINT ( 'NONE',  ( 13.68750000000000178, -0.8284271247459350507, -2.000000000000091926 ) ) ;
#12542=ORIENTED_EDGE ( 'NONE', *, *, #23182, .T. ) ;
#12548=CARTESIAN_POINT ( 'NONE',  ( 18.25000000000009948, 1.110223024625156540E-13, 1.999999999999946265 ) ) ;
#12566=CARTESIAN_POINT ( 'NONE',  ( 0.000000000000000000, 0.000000000000000000, 0.000000000000000000 ) ) ;
#12573=ADVANCED_FACE ( 'NONE', ( #14574 ), #7186, .T. ) ;
#12576=EDGE_CURVE ( 'NONE', #6031, #16041, #16597, .T. ) ;
#12585=AXIS2_PLACEMENT_3D ( 'NONE', #15279, #1879, #20637 ) ;
#12603=CARTESIAN_POINT ( 'NONE',  ( 23.68750000000012790, -0.8284271247461153509, -1.999999999999911626 ) ) ;
#12610=EDGE_LOOP ( 'NONE', ( #7965, #9656, #28962, #27295 ) ) ;
#12617=VECTOR ( 'NONE', #6785, 1000.000000000000000 ) ;
#12620=CARTESIAN_POINT ( 'NONE',  ( 24.71589091039370700, 1.670749105717314498, -1.562495652617925446 ) ) ;
#12631=DIRECTION ( 'NONE',  ( -1.000000000000000000, -1.665334536937731113E-16, 1.526556658859586792E-16 ) ) ;
#12632=CARTESIAN_POINT ( 'NONE',  ( 13.91367513459485039, -1.767766952966209892, -1.767766952966487448 ) ) ;
#12643=CARTESIAN_POINT ( 'NONE',  ( 13.39882486540532724, -1.035533905932629173, -2.499999999999904521 ) ) ;
#12661=CARTESIAN_POINT ( 'NONE',  ( 25.37500000000009237, 2.649519052838500421, -5.551115123125782702E-14 ) ) ;
#12666=CARTESIAN_POINT ( 'NONE',  ( 14.96132486540535567, 5.551115123125782702E-14, 2.500000000000002220 ) ) ;
#12691=CARTESIAN_POINT ( 'NONE',  ( 15.49999999999998579, -1.999999999999835243, 0.000000000000000000 ) ) ;
#12700=CARTESIAN_POINT ( 'NONE',  ( 16.43750000000008527, -1.999999999999851674, 0.8284271247461753029 ) ) ;
#12705=DIRECTION ( 'NONE',  ( -8.326672684688675286E-17, -2.081668171172168821E-17, 1.000000000000000000 ) ) ;
#12742=CARTESIAN_POINT ( 'NONE',  ( 21.28867513459486815, 2.500000000000002220, -1.665334536937734811E-13 ) ) ;
#12756=CARTESIAN_POINT ( 'NONE',  ( 24.87500000000009237, 1.414213562373312083, -1.414213562373145550 ) ) ;
#12760=CARTESIAN_POINT ( 'NONE',  ( 15.96132486540519047, 1.665334536937734811E-13, 2.500000000000057732 ) ) ;
#12763=CARTESIAN_POINT ( 'NONE',  ( 14.81250000000001599, 1.097466725451679892, 2.649519052838298805 ) ) ;
#12781=CARTESIAN_POINT ( 'NONE',  ( 14.06250000000011546, 2.000000000000151879, 0.8284271247461753029 ) ) ;
#12805=CARTESIAN_POINT ( 'NONE',  ( 11.12500000000010658, 1.414213562373201061, 1.414213562373034527 ) ) ;
#12814=CARTESIAN_POINT ( 'NONE',  ( 9.687499999999998224, -0.8284271247461152399, -1.999999999999971800 ) ) ;
#12827=CARTESIAN_POINT ( 'NONE',  ( 24.50000000000010658, 5.586935463532396279E-14, -2.500000000000054623 ) ) ;
#12838=CARTESIAN_POINT ( 'NONE',  ( 15.00000000000012434, 2.000000000000112799, 0.000000000000000000 ) ) ;
#12847=CARTESIAN_POINT ( 'NONE',  ( 16.31250000000011369, -0.8284271247460553989, 1.999999999999971800 ) ) ;
#12848=ORIENTED_EDGE ( 'NONE', *, *, #27785, .F. ) ;
#12852=CARTESIAN_POINT ( 'NONE',  ( 14.56250000000007994, 1.097466725451619718, 2.649519052838298805 ) ) ;
#12862=FILL_AREA_STYLE_COLOUR ( '', #10957 ) ;
#12876=CARTESIAN_POINT ( 'NONE',  ( 21.56250000000015987, -1.999999999999911626, -0.8284271247462354770 ) ) ;
#12877=CARTESIAN_POINT ( 'NONE',  ( 10.46132486540518514, 5.551115123125782702E-14, -2.499999999999946709 ) ) ;
#12900=ORIENTED_EDGE ( 'NONE', *, *, #22570, .F. ) ;
#12902=FACE_OUTER_BOUND ( 'NONE', #9463, .T. ) ;
#12916=CARTESIAN_POINT ( 'NONE',  ( 13.87500000000008171, 1.665334536937734811E-13, 2.649519052838167354 ) ) ;
#12928=ORIENTED_EDGE ( 'NONE', *, *, #16238, .F. ) ;
#12932=( GEOMETRIC_REPRESENTATION_CONTEXT ( 3 ) GLOBAL_UNCERTAINTY_ASSIGNED_CONTEXT ( ( #28447 ) ) GLOBAL_UNIT_ASSIGNED_CONTEXT ( ( #19456, #10703, #22048 ) ) REPRESENTATION_CONTEXT ( 'NONE', 'WORKASPACE' ) );
#12938=CARTESIAN_POINT ( 'NONE',  ( 20.14882486540532014, -2.499999999999964473, 1.035533905932749299 ) ) ;
#12940=CARTESIAN_POINT ( 'NONE',  ( 15.00000000000012434, 2.000000000000112799, 0.000000000000000000 ) ) ;
#12953=COLOUR_RGB ( '', 0.66274510, 0.83137255, 0.94901961) ;
#12970=CARTESIAN_POINT ( 'NONE',  ( 9.562500000000090594, -1.999999999999851674, -0.8284271247462354770 ) ) ;
#12988=FACE_OUTER_BOUND ( 'NONE', #20795, .T. ) ;
#12989=EDGE_LOOP ( 'NONE', ( #11808, #23044, #4005, #25419 ) ) ;
#12993=ORIENTED_EDGE ( 'NONE', *, *, #12094, .F. ) ;
#13004=CARTESIAN_POINT ( 'NONE',  ( 18.06250000000005684, 2.000000000000151879, 0.8284271247461153509 ) ) ;
#13008=CARTESIAN_POINT ( 'NONE',  ( 13.06250000000009948, -1.097466725451499370, -2.649519052838419153 ) ) ;
#13016=SURFACE_STYLE_FILL_AREA ( #26774 ) ;
#13047=CARTESIAN_POINT ( 'NONE',  ( 16.56249999999998934, 1.097466725451619718, 2.649519052838419153 ) ) ;
#13074=CARTESIAN_POINT ( 'NONE',  ( 15.37500000000013856, 1.665334536937734811E-13, -2.649519052838444910 ) ) ;
#13077=EDGE_CURVE ( 'NONE', #12351, #19802, #29199, .T. ) ;
#13084=CARTESIAN_POINT ( 'NONE',  ( 12.03867513459491789, 1.665334536937734811E-13, -2.500000000000057732 ) ) ;
#13086=CARTESIAN_POINT ( 'NONE',  ( 24.91019988680152153, 2.044085285770432137, -0.5010375219942392322 ) ) ;
#13112=CARTESIAN_POINT ( 'NONE',  ( 24.50000000000013145, 1.873492889145067508, -1.873492889145011997 ) ) ;
#13138=CARTESIAN_POINT ( 'NONE',  ( 24.54902502698629618, -0.5994519693307550634, 2.381340238839862788 ) ) ;
#13143=CARTESIAN_POINT ( 'NONE',  ( 10.22617513459487881, 2.500000000000144773, -1.035533905932869425 ) ) ;
#13146=VERTEX_POINT ( 'NONE', #20007 ) ;
#13155=CARTESIAN_POINT ( 'NONE',  ( 14.87500000000011013, 1.414213562373201061, -1.414213562373090038 ) ) ;
#13168=CARTESIAN_POINT ( 'NONE',  ( 16.00000000000007105, 2.000000000000223821, -5.551115123125782702E-14 ) ) ;
#13171=CARTESIAN_POINT ( 'NONE',  ( 13.31250000000003553, 2.649519052838298805, -1.097466725451559322 ) ) ;
#13191=CARTESIAN_POINT ( 'NONE',  ( 22.50000000000010303, -1.999999999999835243, 0.000000000000000000 ) ) ;
#13192=CARTESIAN_POINT ( 'NONE',  ( 10.96132486540515849, 1.110223024625156540E-13, 2.499999999999835687 ) ) ;
#13194=VERTEX_POINT ( 'NONE', #19564 ) ;
#13213=EDGE_CURVE ( 'NONE', #5395, #19802, #22136, .T. ) ;
#13231=ORIENTED_EDGE ( 'NONE', *, *, #5752, .F. ) ;
#13247=CARTESIAN_POINT ( 'NONE',  ( 12.43750000000010836, -1.999999999999851674, 0.8284271247462955401 ) ) ;
#13262=CARTESIAN_POINT ( 'NONE',  ( 23.62500000000011724, 2.649519052838500421, -5.551115123125782702E-14 ) ) ;
#13267=ORIENTED_EDGE ( 'NONE', *, *, #8979, .F. ) ;
#13269=CARTESIAN_POINT ( 'NONE',  ( 15.08632486540523132, -1.767766952966265404, 1.767766952966376426 ) ) ;
#13272=FACE_OUTER_BOUND ( 'NONE', #5089, .T. ) ;
#13281=CARTESIAN_POINT ( 'NONE',  ( 20.93750000000008171, 2.000000000000212275, -0.8284271247463557142 ) ) ;
#13283=ADVANCED_FACE ( 'NONE', ( #6182 ), #10975, .T. ) ;
#13297=SURFACE_STYLE_USAGE ( .BOTH. , #27216 ) ;
#13302=CARTESIAN_POINT ( 'NONE',  ( 13.31250000000012612, -0.8284271247460552878, 1.999999999999911626 ) ) ;
#13305=ORIENTED_EDGE ( 'NONE', *, *, #8979, .T. ) ;
#13309=ORIENTED_EDGE ( 'NONE', *, *, #20609, .T. ) ;
#13313=CARTESIAN_POINT ( 'NONE',  ( 12.25000000000006573, 5.551115123125782702E-14, 1.999999999999946265 ) ) ;
#13314=ORIENTED_EDGE ( 'NONE', *, *, #20609, .F. ) ;
#13316=CARTESIAN_POINT ( 'NONE',  ( 14.37500000000016520, 2.649519052838611444, -5.551115123125782702E-14 ) ) ;
#13341=EDGE_CURVE ( 'NONE', #305, #28521, #30274, .T. ) ;
#13342=CARTESIAN_POINT ( 'NONE',  ( 24.94529002296924602, 1.767886127012007424, -1.055868358531008244 ) ) ;
#13355=VERTEX_POINT ( 'NONE', #11595 ) ;
#13361=CARTESIAN_POINT ( 'NONE',  ( 23.64882486540533435, 2.500000000000084821, -1.035533905932869425 ) ) ;
#13365=CARTESIAN_POINT ( 'NONE',  ( 11.35117513459492322, 2.500000000000084821, 1.035533905932689347 ) ) ;
#13368=CARTESIAN_POINT ( 'NONE',  ( 14.18750000000011369, -2.649519052838298805, -1.097466725451559322 ) ) ;
#13371=CARTESIAN_POINT ( 'NONE',  ( 11.03867513459494454, 1.665334536937734811E-13, -2.500000000000113243 ) ) ;
#13394=CARTESIAN_POINT ( 'NONE',  ( 12.37500000000013500, -1.414213562372979016, 1.414213562373034527 ) ) ;
#13397=CARTESIAN_POINT ( 'NONE',  ( 23.08632486540540540, -1.767766952966209892, 1.767766952966376426 ) ) ;
#13413=CARTESIAN_POINT ( 'NONE',  ( 10.12500000000007816, 1.414213562373201061, 1.414213562373145550 ) ) ;
#13425=CARTESIAN_POINT ( 'NONE',  ( 21.93750000000006395, 2.000000000000212275, -0.8284271247462955401 ) ) ;
#13449=CARTESIAN_POINT ( 'NONE',  ( 13.56250000000003375, -1.999999999999971800, -0.8284271247462354770 ) ) ;
#13454=CARTESIAN_POINT ( 'NONE',  ( 14.14882486540528816, -2.499999999999964473, 1.035533905932749299 ) ) ;
#13457=( BOUNDED_CURVE ( )  B_SPLINE_CURVE ( 2, ( #19815, #3822, #10935, #3359, #17539, #7979, #12632, #3666, #15401 ),
 .UNSPECIFIED., .F., .F. ) 
 B_SPLINE_CURVE_WITH_KNOTS ( ( 3, 2, 2, 2, 3 ),
 ( 0.2343750000000000000, 0.2421875000000000000, 0.2500000000000000000, 0.2578125000000000000, 0.2656250000000000000 ),
 .UNSPECIFIED. ) 
 CURVE ( )  GEOMETRIC_REPRESENTATION_ITEM ( )  RATIONAL_B_SPLINE_CURVE ( ( 1.000000000000000000, 0.9238795325112867385, 1.000000000000000000, 0.9238795325112867385, 1.000000000000000000, 0.9238795325112867385, 1.000000000000000000, 0.9238795325112867385, 1.000000000000000000 ) ) 
 REPRESENTATION_ITEM ( '' )  );
#13460=CARTESIAN_POINT ( 'NONE',  ( 13.00000000000003908, 2.000000000000112799, 0.000000000000000000 ) ) ;
#13469=CARTESIAN_POINT ( 'NONE',  ( 24.49999999999999289, 0.6095397824026904665, 2.424553825690067832 ) ) ;
#13486=CARTESIAN_POINT ( 'NONE',  ( 19.56250000000009948, -1.999999999999911626, -0.8284271247461753029 ) ) ;
#13497=ORIENTED_EDGE ( 'NONE', *, *, #25590, .T. ) ;
#13500=CARTESIAN_POINT ( 'NONE',  ( 17.46132486540527395, 5.551115123125782702E-14, -2.500000000000002220 ) ) ;
#13524=CARTESIAN_POINT ( 'NONE',  ( 11.43750000000000355, 1.097466725451559322, -2.649519052838298805 ) ) ;
#13532=ORIENTED_EDGE ( 'NONE', *, *, #8021, .F. ) ;
#13546=CARTESIAN_POINT ( 'NONE',  ( 12.25000000000006573, 5.551115123125782702E-14, 1.999999999999946265 ) ) ;
#13563=CARTESIAN_POINT ( 'NONE',  ( 22.12500000000006040, -2.649519052838111843, 0.000000000000000000 ) ) ;
#13583=EDGE_CURVE ( 'NONE', #13146, #5962, #26272, .T. ) ;
#13584=CARTESIAN_POINT ( 'NONE',  ( 14.66367513459496053, -1.767766952966320915, 1.767766952966431937 ) ) ;
#13585=CARTESIAN_POINT ( 'NONE',  ( 24.87500000000009237, 1.414213562373312083, -1.414213562373145550 ) ) ;
#13596=CYLINDRICAL_SURFACE ( 'NONE', #12585, 2.499999999999999112 ) ;
#13605=CARTESIAN_POINT ( 'NONE',  ( 12.62500000000013678, -1.414213562372979016, -1.414213562373145550 ) ) ;
#13608=CARTESIAN_POINT ( 'NONE',  ( 14.21132486540527218, -2.499999999999946709, -5.551115123125782702E-14 ) ) ;
#13612=CARTESIAN_POINT ( 'NONE',  ( 11.50000000000006573, -1.999999999999835243, 0.000000000000000000 ) ) ;
#13616=CARTESIAN_POINT ( 'NONE',  ( 18.96132486540530593, 1.110223024625156540E-13, 2.499999999999724665 ) ) ;
#13627=CARTESIAN_POINT ( 'NONE',  ( 22.53867513459501026, 1.110223024625156540E-13, 2.499999999999835687 ) ) ;
#13638=CARTESIAN_POINT ( 'NONE',  ( 20.75000000000012790, 1.665334536937734811E-13, -2.000000000000001776 ) ) ;
#13676=CARTESIAN_POINT ( 'NONE',  ( 11.81250000000017764, 1.097466725451679892, 2.649519052838238409 ) ) ;
#13680=CARTESIAN_POINT ( 'NONE',  ( 23.91367513459499605, -1.767766952966154381, -1.767766952966542959 ) ) ;
#13682=CARTESIAN_POINT ( 'NONE',  ( 12.96132486540529882, 1.110223024625156540E-13, 2.500000000000002220 ) ) ;
#13696=CARTESIAN_POINT ( 'NONE',  ( 22.31250000000008882, 2.649519052838478661, -1.097466725451499370 ) ) ;
#13715=LINE ( 'NONE', #5860, #4481 ) ;
#13721=CARTESIAN_POINT ( 'NONE',  ( 19.81250000000015277, 1.097466725451679892, 2.649519052838298805 ) ) ;
#13723=DIRECTION ( 'NONE',  ( -8.326672684688675286E-17, -2.081668171172168821E-17, 1.000000000000000000 ) ) ;
#13730=CARTESIAN_POINT ( 'NONE',  ( 17.21132486540530238, -2.499999999999891198, -1.110223024625156540E-13 ) ) ;
#13732=ORIENTED_EDGE ( 'NONE', *, *, #15426, .T. ) ;
#13740=CARTESIAN_POINT ( 'NONE',  ( 22.50000000000010303, -1.999999999999835243, 0.000000000000000000 ) ) ;
#13762=CARTESIAN_POINT ( 'NONE',  ( -2.081668171172168020E-16, -5.204170427930420051E-17, 2.499999999999999112 ) ) ;
#13764=CARTESIAN_POINT ( 'NONE',  ( 21.91367513459491079, -1.767766952966154381, -1.767766952966431937 ) ) ;
#13771=CARTESIAN_POINT ( 'NONE',  ( 15.12500000000000000, 1.414213562373201061, 1.414213562373034527 ) ) ;
#13773=VECTOR ( 'NONE', #25975, 1000.000000000000000 ) ;
#13775=CARTESIAN_POINT ( 'NONE',  ( 18.52382486540528461, 1.035533905932869425, -2.499999999999904521 ) ) ;
#13777=CARTESIAN_POINT ( 'NONE',  ( 10.12500000000007816, 1.414213562373201061, 1.414213562373145550 ) ) ;
#13782=SHAPE_DEFINITION_REPRESENTATION ( #3750, #1893 ) ;
#13794=CARTESIAN_POINT ( 'NONE',  ( 10.96132486540515849, 1.110223024625156540E-13, 2.499999999999835687 ) ) ;
#13798=CARTESIAN_POINT ( 'NONE',  ( 20.18750000000014566, 0.8284271247463557142, 1.999999999999911626 ) ) ;
#13808=ORIENTED_EDGE ( 'NONE', *, *, #9688, .F. ) ;
#13809=ADVANCED_FACE ( 'NONE', ( #22093 ), #3035, .T. ) ;
#13810=ORIENTED_EDGE ( 'NONE', *, *, #12576, .T. ) ;
#13814=VERTEX_POINT ( 'NONE', #7944 ) ;
#13833=CARTESIAN_POINT ( 'NONE',  ( 12.06250000000005507, -2.649519052838238409, 1.097466725451619718 ) ) ;
#13836=CARTESIAN_POINT ( 'NONE',  ( 15.97617513459489125, -1.035533905932629173, -2.499999999999964473 ) ) ;
#13839=CARTESIAN_POINT ( 'NONE',  ( 23.72617513459496053, -2.499999999999904521, 1.035533905932749299 ) ) ;
#13853=CARTESIAN_POINT ( 'NONE',  ( 21.81250000000006395, -2.649519052838238409, 1.097466725451499370 ) ) ;
#13860=CARTESIAN_POINT ( 'NONE',  ( 11.06250000000006928, 2.000000000000091926, 0.8284271247461753029 ) ) ;
#13877=CARTESIAN_POINT ( 'NONE',  ( 19.43749999999998224, 1.097466725451559322, -2.649519052838298805 ) ) ;
#13889=CARTESIAN_POINT ( 'NONE',  ( 22.27382486540526330, -2.499999999999904521, -1.035533905932749299 ) ) ;
#13891=CARTESIAN_POINT ( 'NONE',  ( 10.00000000000014744, 1.031164828675704914, 2.068637288563754062 ) ) ;
#13899=CARTESIAN_POINT ( 'NONE',  ( 21.06250000000004619, 2.000000000000151879, 0.8284271247461152399 ) ) ;
#13903=CARTESIAN_POINT ( 'NONE',  ( 11.91367513459487526, -1.767766952966154381, -1.767766952966542959 ) ) ;
#13906=CARTESIAN_POINT ( 'NONE',  ( 24.68421870695930309, -2.320578051741148062, -0.02763398118663714514 ) ) ;
#13928=VECTOR ( 'NONE', #25578, 1000.000000000000000 ) ;
#13929=CARTESIAN_POINT ( 'NONE',  ( 11.37500000000010658, -1.414213562372979016, 1.414213562372979016 ) ) ;
#13957=CARTESIAN_POINT ( 'NONE',  ( 19.87500000000017053, 1.414213562373312083, -1.414213562373145550 ) ) ;
#13959=DIRECTION ( 'NONE',  ( -1.000000000000000000, -1.665334536937731113E-16, 1.526556658859586792E-16 ) ) ;
#13963=( NAMED_UNIT ( * ) PLANE_ANGLE_UNIT ( ) SI_UNIT ( $, .RADIAN. ) );
#13993=CARTESIAN_POINT ( 'NONE',  ( 10.74999999999998224, 1.873492889145123019, 1.873492889144734441 ) ) ;
#13995=CARTESIAN_POINT ( 'NONE',  ( 16.03867513459497474, 5.551115123125782702E-14, -2.500000000000057732 ) ) ;
#14006=CARTESIAN_POINT ( 'NONE',  ( 20.68750000000004974, -1.097466725451439196, 2.649519052838419153 ) ) ;
#14013=CARTESIAN_POINT ( 'NONE',  ( 10.56250000000007461, -1.999999999999971800, -0.8284271247462354770 ) ) ;
#14025=EDGE_CURVE ( 'NONE', #18896, #19610, #10562, .T. ) ;
#14031=ORIENTED_EDGE ( 'NONE', *, *, #14025, .F. ) ;
#14032=CARTESIAN_POINT ( 'NONE',  ( 19.37500000000014211, 1.665334536937734811E-13, -2.649519052838333888 ) ) ;
#14044=CARTESIAN_POINT ( 'NONE',  ( 20.60117513459488237, -1.035533905932568999, 2.499999999999844569 ) ) ;
#14047=CARTESIAN_POINT ( 'NONE',  ( 12.68750000000013500, -1.097466725451379244, 2.649519052838178457 ) ) ;
#14050=CARTESIAN_POINT ( 'NONE',  ( 19.12500000000014211, 1.414213562373256572, 1.414213562373034527 ) ) ;
#14056=CARTESIAN_POINT ( 'NONE',  ( 12.72617513459496408, -2.499999999999964473, 1.035533905932749299 ) ) ;
#14059=CARTESIAN_POINT ( 'NONE',  ( 24.80639502529410834, -0.7518803807380188831, -2.066273979619694501 ) ) ;
#14064=CARTESIAN_POINT ( 'NONE',  ( 15.77382486540523310, 2.500000000000084821, 1.035533905932689347 ) ) ;
#14076=CARTESIAN_POINT ( 'NONE',  ( 11.50000000000006573, -1.999999999999835243, 0.000000000000000000 ) ) ;
#14094=CYLINDRICAL_SURFACE ( 'NONE', #24071, 2.499999999999999112 ) ;
#14131=( GEOMETRIC_REPRESENTATION_CONTEXT ( 3 ) GLOBAL_UNCERTAINTY_ASSIGNED_CONTEXT ( ( #9765 ) ) GLOBAL_UNIT_ASSIGNED_CONTEXT ( ( #8652, #25531, #16366 ) ) REPRESENTATION_CONTEXT ( 'NONE', 'WORKASPACE' ) );
#14132=AXIS2_PLACEMENT_3D ( 'NONE', #8926, #16478, #11718 ) ;
#14145=CARTESIAN_POINT ( 'NONE',  ( 10.12500000000007816, -2.649519052838111843, 1.110223024625156540E-13 ) ) ;
#14149=CARTESIAN_POINT ( 'NONE',  ( 23.78867513459503868, -2.499999999999891198, -2.220446049250313081E-13 ) ) ;
#14154=ORIENTED_EDGE ( 'NONE', *, *, #5857, .T. ) ;
#14159=CARTESIAN_POINT ( 'NONE',  ( 23.37500000000003553, 2.649519052838444910, 0.000000000000000000 ) ) ;
#14181=CARTESIAN_POINT ( 'NONE',  ( 23.12500000000011724, -2.649519052838167354, -1.665334536937734811E-13 ) ) ;
#14200=CARTESIAN_POINT ( 'NONE',  ( 12.75000000000017764, -1.873492889144845464, 1.873492889144845464 ) ) ;
#14205=CARTESIAN_POINT ( 'NONE',  ( 5.000000000000087930, 5.551115123125782702E-14, -5.551115123125782702E-14 ) ) ;
#14207=CYLINDRICAL_SURFACE ( 'NONE', #26854, 2.499999999999999112 ) ;
#14254=EDGE_CURVE ( 'NONE', #22647, #26264, #2132, .T. ) ;
#14264=ADVANCED_FACE ( 'NONE', ( #21546 ), #2631, .T. ) ;
#14265=CARTESIAN_POINT ( 'NONE',  ( 22.93749999999996447, 1.999999999999971800, -0.8284271247462354770 ) ) ;
#14287=ORIENTED_EDGE ( 'NONE', *, *, #20882, .F. ) ;
#14296=CARTESIAN_POINT ( 'NONE',  ( 15.27382486540527040, -2.499999999999844569, -1.035533905932809473 ) ) ;
#14297=CARTESIAN_POINT ( 'NONE',  ( -2.081668171172168020E-16, -5.204170427930420051E-17, 2.499999999999999112 ) ) ;
#14305=CARTESIAN_POINT ( 'NONE',  ( 23.50000000000013145, 1.873492889145011997, 1.873492889144734441 ) ) ;
#14327=CARTESIAN_POINT ( 'NONE',  ( 17.93750000000014921, -1.097466725451439196, 2.649519052838178457 ) ) ;
#14337=ORIENTED_EDGE ( 'NONE', *, *, #2686, .F. ) ;
#14345=CARTESIAN_POINT ( 'NONE',  ( 10.00000000000003730, -1.873492889144789952, -1.873492889145123019 ) ) ;
#14347=CARTESIAN_POINT ( 'NONE',  ( 18.31249999999999289, -0.8284271247460552878, 2.000000000000031530 ) ) ;
#14385=CIRCLE ( 'NONE', #5856, 6.000000000000000888 ) ;
#14405=DIRECTION ( 'NONE',  ( -8.326672684688675286E-17, -2.081668171172168821E-17, 1.000000000000000000 ) ) ;
#14410=ORIENTED_EDGE ( 'NONE', *, *, #13583, .F. ) ;
#14414=CARTESIAN_POINT ( 'NONE',  ( 20.81250000000013856, 0.8284271247461753029, -2.000000000000091926 ) ) ;
#14425=AXIS2_PLACEMENT_3D ( 'NONE', #14205, #5369, #28417 ) ;
#14448=CARTESIAN_POINT ( 'NONE',  ( 17.37500000000000000, 2.649519052838500421, 0.000000000000000000 ) ) ;
#14472=CARTESIAN_POINT ( 'NONE',  ( 16.75000000000001421, 1.873492889145011997, 1.873492889144845464 ) ) ;
#14477=EDGE_LOOP ( 'NONE', ( #8582, #22886, #7448, #8139 ) ) ;
#14485=CARTESIAN_POINT ( 'NONE',  ( 21.03867513459492500, 1.665334536937734811E-13, -2.500000000000002220 ) ) ;
#14489=CARTESIAN_POINT ( 'NONE',  ( 24.02382486540523487, -1.035533905932689347, 2.499999999999964473 ) ) ;
#14493=CARTESIAN_POINT ( 'NONE',  ( 19.43750000000013145, -1.999999999999851674, 0.8284271247462354770 ) ) ;
#14499=CARTESIAN_POINT ( 'NONE',  ( 12.27382486540534146, -2.499999999999784173, -1.035533905932809473 ) ) ;
#14508=( NAMED_UNIT ( * ) PLANE_ANGLE_UNIT ( ) SI_UNIT ( $, .RADIAN. ) );
#14524=ADVANCED_FACE ( 'NONE', ( #20294 ), #8606, .T. ) ;
#14539=CARTESIAN_POINT ( 'NONE',  ( 18.12500000000000355, 1.414213562373090038, 1.414213562373090038 ) ) ;
#14549=CARTESIAN_POINT ( 'NONE',  ( 21.93750000000006395, 2.000000000000212275, -0.8284271247462955401 ) ) ;
#14560=FACE_OUTER_BOUND ( 'NONE', #4021, .T. ) ;
#14568=CARTESIAN_POINT ( 'NONE',  ( 23.56250000000009948, -1.999999999999851674, -0.8284271247462354770 ) ) ;
#14571=CARTESIAN_POINT ( 'NONE',  ( 20.41367513459496763, 1.767766952966487448, 1.767766952966209892 ) ) ;
#14574=FACE_OUTER_BOUND ( 'NONE', #2633, .T. ) ;
#14581=CARTESIAN_POINT ( 'NONE',  ( 18.87500000000011369, -2.649519052838111843, 0.000000000000000000 ) ) ;
#14593=CARTESIAN_POINT ( 'NONE',  ( 15.46132486540530238, 1.110223024625156540E-13, -2.500000000000057732 ) ) ;
#14606=CARTESIAN_POINT ( 'NONE',  ( 19.12500000000003197, -2.649519052838111843, -5.551115123125782702E-14 ) ) ;
#14612=CARTESIAN_POINT ( 'NONE',  ( 23.53867513459495342, 1.665334536937734811E-13, 2.499999999999835687 ) ) ;
#14622=( BOUNDED_CURVE ( )  B_SPLINE_CURVE ( 2, ( #23814, #26399, #2753, #12324, #26548, #21668, #604, #9990, #19366 ),
 .UNSPECIFIED., .F., .F. ) 
 B_SPLINE_CURVE_WITH_KNOTS ( ( 3, 2, 2, 2, 3 ),
 ( 0.1093750000000000000, 0.1171875000000000000, 0.1250000000000000000, 0.1328125000000000000, 0.1406250000000000000 ),
 .UNSPECIFIED. ) 
 CURVE ( )  GEOMETRIC_REPRESENTATION_ITEM ( )  RATIONAL_B_SPLINE_CURVE ( ( 1.000000000000000000, 0.9238795325112867385, 1.000000000000000000, 0.9238795325112867385, 1.000000000000000000, 0.9238795325112867385, 1.000000000000000000, 0.9238795325112867385, 1.000000000000000000 ) ) 
 REPRESENTATION_ITEM ( '' )  );
#14626=CARTESIAN_POINT ( 'NONE',  ( 11.00000000000009237, -1.873492889144900975, -1.873492889145123019 ) ) ;
#14627=CARTESIAN_POINT ( 'NONE',  ( 19.33632486540532014, -1.767766952966265404, -1.767766952966487448 ) ) ;
#14630=CARTESIAN_POINT ( 'NONE',  ( 20.37500000000017053, -1.414213562372979016, 1.414213562373034527 ) ) ;
#14636=DIRECTION ( 'NONE',  ( -1.000000000000000000, -1.665334536937731113E-16, 1.526556658859586792E-16 ) ) ;
#14647=CARTESIAN_POINT ( 'NONE',  ( 11.62499999999999645, -1.414213562373090038, -1.414213562373090038 ) ) ;
#14651=EDGE_CURVE ( 'NONE', #29880, #22647, #15345, .T. ) ;
#14652=CARTESIAN_POINT ( 'NONE',  ( 11.14882486540523843, -2.499999999999964473, 1.035533905932749299 ) ) ;
#14660=CARTESIAN_POINT ( 'NONE',  ( 2.081668171172167281E-16, 3.582034040661430693E-16, -2.499999999999999112 ) ) ;
#14679=CARTESIAN_POINT ( 'NONE',  ( 17.87500000000008527, 1.414213562373312083, -1.414213562373145550 ) ) ;
#14682=EDGE_CURVE ( 'NONE', #20580, #29780, #1578, .T. ) ;
#14688=CARTESIAN_POINT ( 'NONE',  ( 21.62500000000017053, -1.414213562372979016, -1.414213562373090038 ) ) ;
#14714=CARTESIAN_POINT ( 'NONE',  ( 22.75000000000015987, 1.110223024625156540E-13, -2.000000000000168310 ) ) ;
#14717=ADVANCED_FACE ( 'NONE', ( #10903 ), #4395, .T. ) ;
#14726=CARTESIAN_POINT ( 'NONE',  ( 17.43750000000003908, 2.649519052838358757, 1.097466725451379244 ) ) ;
#14751=CARTESIAN_POINT ( 'NONE',  ( 18.50000000000004263, 1.873492889145123019, -1.873492889144956486 ) ) ;
#14759=CARTESIAN_POINT ( 'NONE',  ( 17.41367513459490723, 1.767766952966542959, 1.767766952966320915 ) ) ;
#14761=ORIENTED_EDGE ( 'NONE', *, *, #1691, .T. ) ;
#14772=CARTESIAN_POINT ( 'NONE',  ( 17.31250000000004263, -0.8284271247461152399, 2.000000000000091926 ) ) ;
#14794=APPLICATION_CONTEXT ( 'automotive_design' ) ;
#14830=FACE_OUTER_BOUND ( 'NONE', #24248, .T. ) ;
#14837=CARTESIAN_POINT ( 'NONE',  ( 15.75000000000006928, 2.775557561562891351E-13, -2.000000000000057288 ) ) ;
#14857=CARTESIAN_POINT ( 'NONE',  ( 23.31250000000007461, -0.8284271247460552878, 2.000000000000091926 ) ) ;
#14860=CARTESIAN_POINT ( 'NONE',  ( 20.10117513459495342, 1.035533905932869425, -2.499999999999964473 ) ) ;
#14870=CARTESIAN_POINT ( 'NONE',  ( 19.31250000000007105, 2.649519052838419153, -1.097466725451559322 ) ) ;
#14873=( GEOMETRIC_REPRESENTATION_CONTEXT ( 3 ) GLOBAL_UNCERTAINTY_ASSIGNED_CONTEXT ( ( #28353 ) ) GLOBAL_UNIT_ASSIGNED_CONTEXT ( ( #21236, #5071, #26418 ) ) REPRESENTATION_CONTEXT ( 'NONE', 'WORKASPACE' ) );
#14889=CARTESIAN_POINT ( 'NONE',  ( 24.62500000000012079, -1.414213562372923505, -1.414213562373145550 ) ) ;
#14895=CARTESIAN_POINT ( 'NONE',  ( 19.25000000000009948, -1.873492889144845464, -1.873492889145011997 ) ) ;
#14899=ORIENTED_EDGE ( 'NONE', *, *, #21946, .F. ) ;
#14915=CARTESIAN_POINT ( 'NONE',  ( 19.21132486540538764, -2.499999999999835687, -1.110223024625156540E-13 ) ) ;
#14917=CARTESIAN_POINT ( 'NONE',  ( 14.50000000000012434, -1.999999999999779732, -5.551115123125782702E-14 ) ) ;
#14925=AXIS2_PLACEMENT_3D ( 'NONE', #16365, #4181, #11753 ) ;
#14931=VERTEX_POINT ( 'NONE', #25406 ) ;
#14932=CARTESIAN_POINT ( 'NONE',  ( 13.21132486540532724, -2.499999999999891198, -1.110223024625156540E-13 ) ) ;
#14940=CARTESIAN_POINT ( 'NONE',  ( 10.81250000000001243, 0.8284271247461753029, -2.000000000000091926 ) ) ;
#14959=( BOUNDED_CURVE ( )  B_SPLINE_CURVE ( 2, ( #8570, #27290, #119, #13839, #14149, #7028, #13680, #4572, #25772 ),
 .UNSPECIFIED., .F., .T. ) 
 B_SPLINE_CURVE_WITH_KNOTS ( ( 3, 2, 2, 2, 3 ),
 ( 0.8593750000000000000, 0.8671875000000000000, 0.8750000000000000000, 0.8828125000000000000, 0.8906250000000000000 ),
 .UNSPECIFIED. ) 
 CURVE ( )  GEOMETRIC_REPRESENTATION_ITEM ( )  RATIONAL_B_SPLINE_CURVE ( ( 1.000000000000000000, 0.9238795325112867385, 1.000000000000000000, 0.9238795325112867385, 1.000000000000000000, 0.9238795325112867385, 1.000000000000000000, 0.9238795325112867385, 1.000000000000000000 ) ) 
 REPRESENTATION_ITEM ( '' )  );
#14980=CARTESIAN_POINT ( 'NONE',  ( 15.49999999999998579, -1.999999999999835243, 0.000000000000000000 ) ) ;
#14984=CARTESIAN_POINT ( 'NONE',  ( 13.43750000000000355, 2.649519052838419153, 1.097466725451559322 ) ) ;
#14995=CARTESIAN_POINT ( 'NONE',  ( 19.89882486540532724, 1.035533905932809473, 2.499999999999964473 ) ) ;
#14997=DIRECTION ( 'NONE',  ( -1.000000000000000000, -1.665334536937731113E-16, 1.526556658859586792E-16 ) ) ;
#15005=CARTESIAN_POINT ( 'NONE',  ( 22.06250000000015632, 2.000000000000212275, 0.8284271247461753029 ) ) ;
#15016=CARTESIAN_POINT ( 'NONE',  ( 24.95223159194603468, 1.828742805381509795, -0.9313548736353307600 ) ) ;
#15029=ORIENTED_EDGE ( 'NONE', *, *, #10090, .F. ) ;
#15030=DIRECTION ( 'NONE',  ( -1.000000000000000000, -1.665334536937731113E-16, 1.526556658859586792E-16 ) ) ;
#15032=CYLINDRICAL_SURFACE ( 'NONE', #24584, 2.499999999999999112 ) ;
#15045=CARTESIAN_POINT ( 'NONE',  ( 13.62500000000002665, 2.649519052838444910, -5.551115123125782702E-14 ) ) ;
#15054=VERTEX_POINT ( 'NONE', #13794 ) ;
#15068=CARTESIAN_POINT ( 'NONE',  ( 14.37500000000016520, -1.414213562373034527, 1.414213562372979016 ) ) ;
#15084=CARTESIAN_POINT ( 'NONE',  ( 13.02382486540521001, -1.035533905932629173, 2.499999999999964473 ) ) ;
#15105=CARTESIAN_POINT ( 'NONE',  ( 10.25000000000000888, 5.551115123125782702E-14, 2.000000000000001776 ) ) ;
#15118=CARTESIAN_POINT ( 'NONE',  ( 10.46132486540518514, 5.551115123125782702E-14, -2.499999999999946709 ) ) ;
#15122=AXIS2_PLACEMENT_3D ( 'NONE', #19906, #6529, #20229 ) ;
#15128=CARTESIAN_POINT ( 'NONE',  ( 14.06250000000011546, 2.000000000000151879, 0.8284271247461753029 ) ) ;
#15138=CARTESIAN_POINT ( 'NONE',  ( 17.50000000000007105, -1.999999999999835243, -5.551115123125782702E-14 ) ) ;
#15149=PRESENTATION_STYLE_ASSIGNMENT (( #5741 ) ) ;
#15159=DIRECTION ( 'NONE',  ( -8.326672684688675286E-17, -2.081668171172168821E-17, 1.000000000000000000 ) ) ;
#15162=CARTESIAN_POINT ( 'NONE',  ( 17.96132486540527751, 1.110223024625156540E-13, 2.499999999999946709 ) ) ;
#15176=ORIENTED_EDGE ( 'NONE', *, *, #28913, .F. ) ;
#15195=CARTESIAN_POINT ( 'NONE',  ( 25.00000000000013500, 2.000000000000279332, -5.551115123125782702E-14 ) ) ;
#15204=CARTESIAN_POINT ( 'NONE',  ( 16.18750000000005684, -2.649519052838298805, -1.097466725451499370 ) ) ;
#15215=AXIS2_PLACEMENT_3D ( 'NONE', #8086, #1028, #26232 ) ;
#15227=CARTESIAN_POINT ( 'NONE',  ( 16.12500000000002842, 1.414213562373201061, 1.414213562373034527 ) ) ;
#15244=CARTESIAN_POINT ( 'NONE',  ( 24.37500000000006395, 1.110223024625156540E-13, -2.649519052838278377 ) ) ;
#15250=ORIENTED_EDGE ( 'NONE', *, *, #1691, .F. ) ;
#15253=CARTESIAN_POINT ( 'NONE',  ( 10.25000000000000888, 5.551115123125782702E-14, 2.000000000000001776 ) ) ;
#15261=AXIS2_PLACEMENT_3D ( 'NONE', #18029, #20448, #11423 ) ;
#15263=CARTESIAN_POINT ( 'NONE',  ( 24.75000000000015987, -1.873492889144789952, 1.873492889144845464 ) ) ;
#15270=VECTOR ( 'NONE', #11882, 1000.000000000000000 ) ;
#15278=CARTESIAN_POINT ( 'NONE',  ( 10.03867513459497118, 1.110223024625156540E-13, -2.500000000000113243 ) ) ;
#15279=CARTESIAN_POINT ( 'NONE',  ( 0.000000000000000000, 0.000000000000000000, 0.000000000000000000 ) ) ;
#15280=ORIENTED_EDGE ( 'NONE', *, *, #6999, .T. ) ;
#15290=CARTESIAN_POINT ( 'NONE',  ( 14.75000000000009592, 2.220446049250313081E-13, -2.000000000000057288 ) ) ;
#15302=CARTESIAN_POINT ( 'NONE',  ( 17.12500000000005684, 1.414213562373090038, 1.414213562373201061 ) ) ;
#15308=CARTESIAN_POINT ( 'NONE',  ( 15.25000000000001421, 1.873492889145067508, -1.873492889144956486 ) ) ;
#15314=DIRECTION ( 'NONE',  ( -1.000000000000000000, -1.665334536937731113E-16, 1.526556658859586792E-16 ) ) ;
#15345=( BOUNDED_CURVE ( )  B_SPLINE_CURVE ( 2, ( #9826, #26677, #24534, #28533, #26240, #5193, #8093, #19357, #12760 ),
 .UNSPECIFIED., .F., .T. ) 
 B_SPLINE_CURVE_WITH_KNOTS ( ( 3, 2, 2, 2, 3 ),
 ( 0.5156250000000000000, 0.5234375000000000000, 0.5312500000000000000, 0.5390625000000000000, 0.5468750000000000000 ),
 .UNSPECIFIED. ) 
 CURVE ( )  GEOMETRIC_REPRESENTATION_ITEM ( )  RATIONAL_B_SPLINE_CURVE ( ( 1.000000000000000000, 0.9238795325112867385, 1.000000000000000000, 0.9238795325112867385, 1.000000000000000000, 0.9238795325112867385, 1.000000000000000000, 0.9238795325112867385, 1.000000000000000000 ) ) 
 REPRESENTATION_ITEM ( '' )  );
#15350=DIRECTION ( 'NONE',  ( -1.000000000000000000, -1.665334536937731113E-16, 1.526556658859586792E-16 ) ) ;
#15372=CARTESIAN_POINT ( 'NONE',  ( 15.00000000000006928, -1.873492889144900975, 1.873492889144900975 ) ) ;
#15396=CARTESIAN_POINT ( 'NONE',  ( 16.43750000000008527, -1.999999999999851674, 0.8284271247461753029 ) ) ;
#15401=CARTESIAN_POINT ( 'NONE',  ( 14.03867513459489125, 5.551115123125782702E-14, -2.500000000000057732 ) ) ;
#15426=EDGE_CURVE ( 'NONE', #29417, #305, #26699, .T. ) ;
#15427=CARTESIAN_POINT ( 'NONE',  ( 24.37500000000009237, 2.649519052838555933, 5.551115123125782702E-14 ) ) ;
#15428=AXIS2_PLACEMENT_3D ( 'NONE', #12566, #14997, #24337 ) ;
#15443=CARTESIAN_POINT ( 'NONE',  ( 16.03867513459497474, 5.551115123125782702E-14, -2.500000000000057732 ) ) ;
#15453=CARTESIAN_POINT ( 'NONE',  ( 13.87500000000011013, 1.414213562373312083, -1.414213562373145550 ) ) ;
#15464=CARTESIAN_POINT ( 'NONE',  ( 17.68750000000009592, -0.8284271247460553989, -1.999999999999971800 ) ) ;
#15486=CARTESIAN_POINT ( 'NONE',  ( 22.31250000000002842, -0.8284271247460552878, 2.000000000000031530 ) ) ;
#15509=CARTESIAN_POINT ( 'NONE',  ( 0.000000000000000000, 0.000000000000000000, 0.000000000000000000 ) ) ;
#15516=CARTESIAN_POINT ( 'NONE',  ( 23.83632486540529527, 1.767766952966487448, 1.767766952966320915 ) ) ;
#15524=CARTESIAN_POINT ( 'NONE',  ( 14.93749999999998401, -1.097466725451499370, 2.649519052838298805 ) ) ;
#15536=ORIENTED_EDGE ( 'NONE', *, *, #6053, .T. ) ;
#15551=CARTESIAN_POINT ( 'NONE',  ( 12.50000000000012257, -1.999999999999835243, 0.000000000000000000 ) ) ;
#15570=CARTESIAN_POINT ( 'NONE',  ( 16.52382486540528106, 1.035533905932929599, -2.500000000000024425 ) ) ;
#15580=CARTESIAN_POINT ( 'NONE',  ( 10.00000000000014744, 1.428066816532635119, 1.737247053690839760 ) ) ;
#15611=CARTESIAN_POINT ( 'NONE',  ( 13.62500000000016520, -1.414213562372923505, -1.414213562373145550 ) ) ;
#15621=CARTESIAN_POINT ( 'NONE',  ( 11.18750000000003730, 0.8284271247462955401, 2.000000000000031530 ) ) ;
#15624=CARTESIAN_POINT ( 'NONE',  ( 14.50000000000006750, 1.873492889145123019, 1.873492889144845464 ) ) ;
#15632=CARTESIAN_POINT ( 'NONE',  ( 17.52382486540523843, 1.035533905932869425, -2.499999999999904521 ) ) ;
#15672=CARTESIAN_POINT ( 'NONE',  ( 13.47617513459483263, 1.035533905932869425, 2.499999999999844569 ) ) ;
#15680=CARTESIAN_POINT ( 'NONE',  ( 16.00000000000012434, -1.873492889144845464, 1.873492889144845464 ) ) ;
#15701=CARTESIAN_POINT ( 'NONE',  ( 20.46132486540533435, 1.110223024625156540E-13, -2.500000000000057732 ) ) ;
#15702=EDGE_CURVE ( 'NONE', #5319, #24536, #17849, .T. ) ;
#15704=CARTESIAN_POINT ( 'NONE',  ( 11.87500000000007994, 1.414213562373312083, -1.414213562373090038 ) ) ;
#15708=CARTESIAN_POINT ( 'NONE',  ( 23.27382486540533790, -2.499999999999844569, -1.035533905932809473 ) ) ;
#15717=( BOUNDED_CURVE ( )  B_SPLINE_CURVE ( 2, ( #29096, #2745, #21061, #16631, #996, #9832, #8055, #19206, #15162 ),
 .UNSPECIFIED., .F., .F. ) 
 B_SPLINE_CURVE_WITH_KNOTS ( ( 3, 2, 2, 2, 3 ),
 ( 0.3906250000000000000, 0.3984375000000000000, 0.4062500000000000000, 0.4140625000000000000, 0.4218750000000000000 ),
 .UNSPECIFIED. ) 
 CURVE ( )  GEOMETRIC_REPRESENTATION_ITEM ( )  RATIONAL_B_SPLINE_CURVE ( ( 1.000000000000000000, 0.9238795325112867385, 1.000000000000000000, 0.9238795325112867385, 1.000000000000000000, 0.9238795325112867385, 1.000000000000000000, 0.9238795325112867385, 1.000000000000000000 ) ) 
 REPRESENTATION_ITEM ( '' )  );
#15721=ORIENTED_EDGE ( 'NONE', *, *, #9505, .T. ) ;
#15730=CARTESIAN_POINT ( 'NONE',  ( 10.00000000000014744, 0.2433462418246987169, 2.400232754357976450 ) ) ;
#15735=ORIENTED_EDGE ( 'NONE', *, *, #5725, .T. ) ;
#15740=CARTESIAN_POINT ( 'NONE',  ( 23.06250000000011013, 2.000000000000151879, 0.8284271247462354770 ) ) ;
#15750=CARTESIAN_POINT ( 'NONE',  ( 17.03867513459494987, 1.665334536937734811E-13, -2.500000000000002220 ) ) ;
#15776=CARTESIAN_POINT ( 'NONE',  ( 12.81250000000004441, 0.8284271247461753029, -2.000000000000091926 ) ) ;
#15831=CARTESIAN_POINT ( 'NONE',  ( 23.96132486540522422, 5.551115123125782702E-14, 2.500000000000002220 ) ) ;
#15835=DIRECTION ( 'NONE',  ( 0.000000000000000000, -2.081668171172248016E-17, 1.000000000000000000 ) ) ;
#15838=CARTESIAN_POINT ( 'NONE',  ( 12.81250000000010303, 1.097466725451559322, 2.649519052838238409 ) ) ;
#15856=ORIENTED_EDGE ( 'NONE', *, *, #10236, .F. ) ;
#15888=CARTESIAN_POINT ( 'NONE',  ( 10.00000000000014744, 1.172613085279341938, 1.967453276497120429 ) ) ;
#15897=CARTESIAN_POINT ( 'NONE',  ( 19.03867513459492500, 1.110223024625156540E-13, -2.500000000000057732 ) ) ;
#15899=CARTESIAN_POINT ( 'NONE',  ( 22.25000000000010303, 1.110223024625156540E-13, 1.999999999999946265 ) ) ;
#15918=ORIENTED_EDGE ( 'NONE', *, *, #9361, .T. ) ;
#15930=CARTESIAN_POINT ( 'NONE',  ( 14.93750000000010303, 2.000000000000151879, -0.8284271247462955401 ) ) ;
#15931=ORIENTED_EDGE ( 'NONE', *, *, #19252, .T. ) ;
#15933=CARTESIAN_POINT ( 'NONE',  ( 10.00000000000014566, 1.542760454755543353, -1.608875422785432052 ) ) ;
#15936=CARTESIAN_POINT ( 'NONE',  ( 14.03867513459489125, 5.551115123125782702E-14, -2.500000000000057732 ) ) ;
#15940=DIRECTION ( 'NONE',  ( -1.000000000000000000, -1.665334536937731113E-16, 1.526556658859586792E-16 ) ) ;
#15949=CARTESIAN_POINT ( 'NONE',  ( 18.81250000000011013, 0.8284271247462354770, -2.000000000000091926 ) ) ;
#15955=EDGE_LOOP ( 'NONE', ( #5641, #20327, #2044, #4421 ) ) ;
#15957=CARTESIAN_POINT ( 'NONE',  ( 14.64882486540525086, 2.500000000000144773, -1.035533905932749299 ) ) ;
#15984=CARTESIAN_POINT ( 'NONE',  ( 13.00000000000009415, -1.873492889144789952, 1.873492889144845464 ) ) ;
#16003=CARTESIAN_POINT ( 'NONE',  ( 22.00000000000007461, -1.873492889144678930, -1.873492889145011997 ) ) ;
#16011=CARTESIAN_POINT ( 'NONE',  ( 12.00000000000012079, 2.000000000000112799, -1.665334536937734811E-13 ) ) ;
#16014=CARTESIAN_POINT ( 'NONE',  ( 10.00000000000014744, 1.110223024625156540E-13, -5.551115123125782702E-14 ) ) ;
#16018=ADVANCED_FACE ( 'NONE', ( #22198 ), #10531, .T. ) ;
#16029=CARTESIAN_POINT ( 'NONE',  ( 19.62500000000008527, 2.649519052838500421, -5.551115123125782702E-14 ) ) ;
#16031=CARTESIAN_POINT ( 'NONE',  ( 0.000000000000000000, 0.000000000000000000, 0.000000000000000000 ) ) ;
#16041=VERTEX_POINT ( 'NONE', #28931 ) ;
#16049=CARTESIAN_POINT ( 'NONE',  ( 14.60117513459484861, -1.035533905932629173, 2.499999999999784173 ) ) ;
#16050=CARTESIAN_POINT ( 'NONE',  ( 21.25000000000015632, 0.000000000000000000, 2.000000000000057288 ) ) ;
#16055=CARTESIAN_POINT ( 'NONE',  ( 11.97617513459491612, -1.035533905932629173, -2.499999999999964473 ) ) ;
#16060=CARTESIAN_POINT ( 'NONE',  ( 12.28867513459488947, 2.500000000000113243, -1.110223024625156540E-13 ) ) ;
#16080=CARTESIAN_POINT ( 'NONE',  ( 12.12500000000005329, 1.414213562373201061, 1.414213562373034527 ) ) ;
#16081=ORIENTED_EDGE ( 'NONE', *, *, #17850, .F. ) ;
#16084=CARTESIAN_POINT ( 'NONE',  ( 10.25000000000000888, 5.551115123125782702E-14, 2.000000000000001776 ) ) ;
#16107=CARTESIAN_POINT ( 'NONE',  ( 19.50000000000009948, -1.999999999999835243, 0.000000000000000000 ) ) ;
#16116=ORIENTED_EDGE ( 'NONE', *, *, #473, .F. ) ;
#16122=CARTESIAN_POINT ( 'NONE',  ( -2.081668171172168020E-16, -5.204170427930420051E-17, 2.499999999999999112 ) ) ;
#16128=CARTESIAN_POINT ( 'NONE',  ( 23.22617513459493921, 2.500000000000205169, -1.035533905932869425 ) ) ;
#16139=CARTESIAN_POINT ( 'NONE',  ( 12.18750000000011369, -2.649519052838238409, -1.097466725451559322 ) ) ;
#16153=CARTESIAN_POINT ( 'NONE',  ( 23.62500000000017408, 1.110223024625156540E-13, 2.649519052838167354 ) ) ;
#16163=CARTESIAN_POINT ( 'NONE',  ( 11.43750000000003197, -1.999999999999911626, 0.8284271247462955401 ) ) ;
#16166=ADVANCED_FACE ( 'NONE', ( #18172 ), #9230, .T. ) ;
#16181=CARTESIAN_POINT ( 'NONE',  ( 20.93750000000008171, -1.097466725451379244, 2.649519052838178457 ) ) ;
#16188=CARTESIAN_POINT ( 'NONE',  ( 22.46132486540528106, 1.665334536937734811E-13, -2.500000000000113243 ) ) ;
#16189=CARTESIAN_POINT ( 'NONE',  ( 0.000000000000000000, 0.000000000000000000, 0.000000000000000000 ) ) ;
#16191=ORIENTED_EDGE ( 'NONE', *, *, #14254, .T. ) ;
#16198=CARTESIAN_POINT ( 'NONE',  ( 22.93749999999995737, 1.999999999999971800, -0.8284271247462354770 ) ) ;
#16204=CARTESIAN_POINT ( 'NONE',  ( 11.60117513459491967, -1.035533905932568999, 2.499999999999784173 ) ) ;
#16207=CARTESIAN_POINT ( 'NONE',  ( 24.73102515769420506, -2.036758492458766057, -1.044594274058695316 ) ) ;
#16210=VECTOR ( 'NONE', #23717, 1000.000000000000000 ) ;
#16223=CARTESIAN_POINT ( 'NONE',  ( 12.68750000000013500, -0.8284271247459952248, -1.999999999999911626 ) ) ;
#16228=ADVANCED_FACE ( 'NONE', ( #13272 ), #2015, .T. ) ;
#16233=CARTESIAN_POINT ( 'NONE',  ( 11.81250000000005862, 0.8284271247463557142, -2.000000000000031530 ) ) ;
#16238=EDGE_CURVE ( 'NONE', #19610, #14931, #1275, .T. ) ;
#16265=CARTESIAN_POINT ( 'NONE',  ( 14.96132486540535567, 5.551115123125782702E-14, 2.500000000000002220 ) ) ;
#16288=CARTESIAN_POINT ( 'NONE',  ( 21.14882486540530593, -2.499999999999904521, 1.035533905932629173 ) ) ;
#16294=CARTESIAN_POINT ( 'NONE',  ( 12.75000000000009415, 1.873492889145067508, 1.873492889144900975 ) ) ;
#16300=ORIENTED_EDGE ( 'NONE', *, *, #10236, .T. ) ;
#16306=ORIENTED_EDGE ( 'NONE', *, *, #27454, .F. ) ;
#16316=VECTOR ( 'NONE', #12631, 1000.000000000000000 ) ;
#16331=CARTESIAN_POINT ( 'NONE',  ( 22.25000000000015987, -1.873492889144789952, -1.873492889145178530 ) ) ;
#16340=CARTESIAN_POINT ( 'NONE',  ( 17.46132486540527395, 5.551115123125782702E-14, -2.500000000000002220 ) ) ;
#16344=ORIENTED_EDGE ( 'NONE', *, *, #9244, .F. ) ;
#16349=CARTESIAN_POINT ( 'NONE',  ( 10.18750000000011013, 1.097466725451679892, -2.649519052838419153 ) ) ;
#16350=CARTESIAN_POINT ( 'NONE',  ( 14.91367513459485039, -1.767766952966265404, -1.767766952966320915 ) ) ;
#16351=CARTESIAN_POINT ( 'NONE',  ( 21.00000000000007461, 2.000000000000057288, 0.000000000000000000 ) ) ;
#16358=DIRECTION ( 'NONE',  ( -8.326672684688675286E-17, -2.081668171172168821E-17, 1.000000000000000000 ) ) ;
#16365=CARTESIAN_POINT ( 'NONE',  ( 0.000000000000000000, 0.000000000000000000, 0.000000000000000000 ) ) ;
#16366=( NAMED_UNIT ( * ) SI_UNIT ( $, .STERADIAN. ) SOLID_ANGLE_UNIT ( ) );
#16371=LINE ( 'NONE', #13762, #19975 ) ;
#16381=CARTESIAN_POINT ( 'NONE',  ( 10.00000000000014566, 1.739457083235398827, -1.326893112237951700 ) ) ;
#16399=( GEOMETRIC_REPRESENTATION_CONTEXT ( 3 ) GLOBAL_UNCERTAINTY_ASSIGNED_CONTEXT ( ( #115 ) ) GLOBAL_UNIT_ASSIGNED_CONTEXT ( ( #12056, #12209, #2782 ) ) REPRESENTATION_CONTEXT ( 'NONE', 'WORKASPACE' ) );
#16406=CARTESIAN_POINT ( 'NONE',  ( 19.75000000000009948, 1.665334536937734811E-13, -2.000000000000001776 ) ) ;
#16414=FACE_OUTER_BOUND ( 'NONE', #6665, .T. ) ;
#16441=CARTESIAN_POINT ( 'NONE',  ( 10.37500000000013500, 1.665334536937734811E-13, -2.649519052838444910 ) ) ;
#16456=CARTESIAN_POINT ( 'NONE',  ( 20.81250000000017053, -2.649519052838178457, 1.097466725451499370 ) ) ;
#16476=CARTESIAN_POINT ( 'NONE',  ( 20.81250000000014211, 1.097466725451679892, 2.649519052838298805 ) ) ;
#16478=DIRECTION ( 'NONE',  ( -1.000000000000000000, -1.665334536937731113E-16, 1.526556658859586792E-16 ) ) ;
#16484=DIRECTION ( 'NONE',  ( 0.000000000000000000, -2.081668171172247091E-17, 1.000000000000000000 ) ) ;
#16496=CARTESIAN_POINT ( 'NONE',  ( 11.87500000000013500, -2.649519052838111843, 1.110223024625156540E-13 ) ) ;
#16497=DIRECTION ( 'NONE',  ( 0.000000000000000000, -2.081668171172248016E-17, 1.000000000000000000 ) ) ;
#16498=CARTESIAN_POINT ( 'NONE',  ( 17.75000000000015632, 1.110223024625156540E-13, -2.000000000000001776 ) ) ;
#16507=CARTESIAN_POINT ( 'NONE',  ( 24.61237180318302364, -1.845499441024646803, 1.545370191226289602 ) ) ;
#16508=DIRECTION ( 'NONE',  ( -1.000000000000000000, -1.665334536937731113E-16, 1.526556658859586792E-16 ) ) ;
#16556=CARTESIAN_POINT ( 'NONE',  ( 17.50000000000007105, -1.999999999999835243, -5.551115123125782702E-14 ) ) ;
#16564=CARTESIAN_POINT ( 'NONE',  ( 22.56250000000011724, -1.999999999999851674, -0.8284271247462354770 ) ) ;
#16579=CARTESIAN_POINT ( 'NONE',  ( 23.28867513459498184, 2.500000000000113243, -2.220446049250313081E-13 ) ) ;
#16587=CARTESIAN_POINT ( 'NONE',  ( 13.89882486540516915, 1.035533905932809473, 2.499999999999964473 ) ) ;
#16596=CARTESIAN_POINT ( 'NONE',  ( 15.39882486540520823, -1.035533905932568999, -2.500000000000024425 ) ) ;
#16597=LINE ( 'NONE', #14297, #1524 ) ;
#16605=CARTESIAN_POINT ( 'NONE',  ( 22.62500000000011724, 5.551115123125782702E-14, 2.649519052838333888 ) ) ;
#16619=CARTESIAN_POINT ( 'NONE',  ( -4.996003610813206404E-16, -1.249000902703301601E-16, 6.000000000000001776 ) ) ;
#16628=CARTESIAN_POINT ( 'NONE',  ( 21.81250000000003908, 1.097466725451619718, 2.649519052838358757 ) ) ;
#16631=CARTESIAN_POINT ( 'NONE',  ( 18.27382486540526330, -2.499999999999844569, -1.035533905932809473 ) ) ;
#16649=CARTESIAN_POINT ( 'NONE',  ( 19.62500000000008527, -1.414213562372979016, -1.414213562373145550 ) ) ;
#16652=CARTESIAN_POINT ( 'NONE',  ( 2.081668171172167281E-16, 3.582034040661430693E-16, -2.499999999999999112 ) ) ;
#16655=SURFACE_SIDE_STYLE ('',( #7825 ) ) ;
#16656=CARTESIAN_POINT ( 'NONE',  ( 24.71049160502954223, -2.207904618590463386, -0.6243674924216627842 ) ) ;
#16661=ORIENTED_EDGE ( 'NONE', *, *, #11223, .F. ) ;
#16694=CARTESIAN_POINT ( 'NONE',  ( 13.33632486540539652, -1.767766952966320915, -1.767766952966542959 ) ) ;
#16712=CARTESIAN_POINT ( 'NONE',  ( 19.68750000000015632, -0.8284271247461153509, -1.999999999999971800 ) ) ;
#16725=VECTOR ( 'NONE', #10932, 1000.000000000000000 ) ;
#16744=CIRCLE ( 'NONE', #27489, 2.499999999999999112 ) ;
#16747=EDGE_CURVE ( 'NONE', #7693, #1194, #5067, .T. ) ;
#16750=CARTESIAN_POINT ( 'NONE',  ( 17.62500000000005684, 5.551115123125782702E-14, 2.649519052838333888 ) ) ;
#16775=CARTESIAN_POINT ( 'NONE',  ( 16.93750000000007816, -1.097466725451499370, 2.649519052838178457 ) ) ;
#16790=( BOUNDED_CURVE ( )  B_SPLINE_CURVE ( 2, ( #8009, #17416, #26730, #5695, #25195, #11580, #20775, #11431, #15897 ),
 .UNSPECIFIED., .F., .T. ) 
 B_SPLINE_CURVE_WITH_KNOTS ( ( 3, 2, 2, 2, 3 ),
 ( 0.5468750000000000000, 0.5546875000000000000, 0.5625000000000000000, 0.5703125000000000000, 0.5781250000000000000 ),
 .UNSPECIFIED. ) 
 CURVE ( )  GEOMETRIC_REPRESENTATION_ITEM ( )  RATIONAL_B_SPLINE_CURVE ( ( 1.000000000000000000, 0.9238795325112867385, 1.000000000000000000, 0.9238795325112867385, 1.000000000000000000, 0.9238795325112867385, 1.000000000000000000, 0.9238795325112867385, 1.000000000000000000 ) ) 
 REPRESENTATION_ITEM ( '' )  );
#16791=VERTEX_POINT ( 'NONE', #29241 ) ;
#16793=CARTESIAN_POINT ( 'NONE',  ( 24.33632486540526685, -1.767766952966209892, -1.767766952966487448 ) ) ;
#16798=CARTESIAN_POINT ( 'NONE',  ( 17.50000000000007105, -1.999999999999835243, -5.551115123125782702E-14 ) ) ;
#16801=LINE ( 'NONE', #16652, #13773 ) ;
#16805=CARTESIAN_POINT ( 'NONE',  ( 15.41367513459490723, 1.767766952966431937, 1.767766952966209892 ) ) ;
#16806=CARTESIAN_POINT ( 'NONE',  ( 24.81367708707497144, -0.6026874312555234869, -2.107048546424427737 ) ) ;
#16845=CARTESIAN_POINT ( 'NONE',  ( 16.93750000000001421, 2.000000000000151879, -0.8284271247462354770 ) ) ;
#16857=CARTESIAN_POINT ( 'NONE',  ( 20.56250000000014211, -1.999999999999911626, -0.8284271247462354770 ) ) ;
#16876=CARTESIAN_POINT ( 'NONE',  ( 24.22617513459492145, 2.500000000000205169, -1.035533905932869425 ) ) ;
#16879=CARTESIAN_POINT ( 'NONE',  ( 13.52382486540523310, 1.035533905932809473, -2.499999999999904521 ) ) ;
#16883=CARTESIAN_POINT ( 'NONE',  ( 9.125000000000049738, -2.649519052838111843, 0.000000000000000000 ) ) ;
#16886=CARTESIAN_POINT ( 'NONE',  ( 20.16367513459488237, 1.767766952966376426, -1.767766952966431937 ) ) ;
#16894=CARTESIAN_POINT ( 'NONE',  ( 19.93750000000006040, -2.649519052838178457, -1.097466725451619718 ) ) ;
#16917=CARTESIAN_POINT ( 'NONE',  ( 16.68750000000004974, 2.649519052838478661, 1.097466725451499370 ) ) ;
#16926=CARTESIAN_POINT ( 'NONE',  ( 22.35117513459491789, 2.500000000000024425, 1.035533905932689347 ) ) ;
#16933=CARTESIAN_POINT ( 'NONE',  ( 12.43750000000007816, 2.649519052838478661, 1.097466725451439196 ) ) ;
#16937=CARTESIAN_POINT ( 'NONE',  ( 20.25000000000015632, 1.110223024625156540E-13, 1.999999999999946265 ) ) ;
#16941=CARTESIAN_POINT ( 'NONE',  ( 12.14882486540528284, -2.499999999999964473, 1.035533905932749299 ) ) ;
#16942=CARTESIAN_POINT ( 'NONE',  ( 15.22617513459492855, 2.500000000000084821, -1.035533905932929599 ) ) ;
#16960=( BOUNDED_CURVE ( )  B_SPLINE_CURVE ( 2, ( #1232, #8302, #3688, #1393, #10804, #25659, #27792, #4610, #11572 ),
 .UNSPECIFIED., .F., .F. ) 
 B_SPLINE_CURVE_WITH_KNOTS ( ( 3, 2, 2, 2, 3 ),
 ( 0.6093750000000000000, 0.6171875000000000000, 0.6250000000000000000, 0.6328125000000000000, 0.6406250000000000000 ),
 .UNSPECIFIED. ) 
 CURVE ( )  GEOMETRIC_REPRESENTATION_ITEM ( )  RATIONAL_B_SPLINE_CURVE ( ( 1.000000000000000000, 0.9238795325112867385, 1.000000000000000000, 0.9238795325112867385, 1.000000000000000000, 0.9238795325112867385, 1.000000000000000000, 0.9238795325112867385, 1.000000000000000000 ) ) 
 REPRESENTATION_ITEM ( '' )  );
#16991=CARTESIAN_POINT ( 'NONE',  ( 17.68750000000009592, -0.8284271247460552878, -1.999999999999971800 ) ) ;
#16999=CARTESIAN_POINT ( 'NONE',  ( 19.62500000000008527, -1.414213562372979016, -1.414213562373145550 ) ) ;
#17000=ORIENTED_EDGE ( 'NONE', *, *, #22400, .F. ) ;
#17023=CARTESIAN_POINT ( 'NONE',  ( 23.12500000000003553, 1.414213562373090038, 1.414213562373034527 ) ) ;
#17027=CARTESIAN_POINT ( 'NONE',  ( 20.35117513459494631, 2.500000000000205169, 1.035533905932689347 ) ) ;
#17036=CARTESIAN_POINT ( 'NONE',  ( 20.06250000000018474, -1.097466725451379244, -2.649519052838419153 ) ) ;
#17043=LINE ( 'NONE', #7200, #22375 ) ;
#17063=CARTESIAN_POINT ( 'NONE',  ( 18.68749999999999645, 2.649519052838298805, 1.097466725451499370 ) ) ;
#17068=CARTESIAN_POINT ( 'NONE',  ( 17.47617513459483618, 1.035533905932809473, 2.499999999999964473 ) ) ;
#17078=EDGE_CURVE ( 'NONE', #1574, #12351, #7846, .T. ) ;
#17086=CARTESIAN_POINT ( 'NONE',  ( 15.93749999999996980, 2.000000000000091926, -0.8284271247462955401 ) ) ;
#17105=FILL_AREA_STYLE_COLOUR ( '', #8045 ) ;
#17108=CARTESIAN_POINT ( 'NONE',  ( 11.02382486540524020, -1.035533905932689347, 2.499999999999964473 ) ) ;
#17110=ORIENTED_EDGE ( 'NONE', *, *, #532, .F. ) ;
#17111=CARTESIAN_POINT ( 'NONE',  ( 24.03867513459490013, 1.665334536937734811E-13, -2.500000000000002220 ) ) ;
#17114=CARTESIAN_POINT ( 'NONE',  ( 10.00000000000009237, 2.000000000000112799, 0.000000000000000000 ) ) ;
#17144=CARTESIAN_POINT ( 'NONE',  ( 14.46132486540527218, 5.551115123125782702E-14, -2.500000000000057732 ) ) ;
#17148=CARTESIAN_POINT ( 'NONE',  ( 21.31250000000010658, -0.8284271247460553989, 1.999999999999971800 ) ) ;
#17152=CARTESIAN_POINT ( 'NONE',  ( 15.62500000000011013, 1.665334536937734811E-13, 2.649519052838278377 ) ) ;
#17169=CARTESIAN_POINT ( 'NONE',  ( 9.437500000000122569, 1.097466725451679892, -2.649519052838238409 ) ) ;
#17189=CARTESIAN_POINT ( 'NONE',  ( 19.50000000000004619, 1.873492889145178530, 1.873492889144789952 ) ) ;
#17195=CARTESIAN_POINT ( 'NONE',  ( 21.16367513459491079, 1.767766952966542959, -1.767766952966598470 ) ) ;
#17210=CARTESIAN_POINT ( 'NONE',  ( 17.81250000000006395, 1.097466725451619718, 2.649519052838298805 ) ) ;
#17223=CARTESIAN_POINT ( 'NONE',  ( 24.53846405162355993, 0.8441100269167298720, -2.325921235098170836 ) ) ;
#17229=CARTESIAN_POINT ( 'NONE',  ( 10.68750000000004441, -0.8284271247460553989, -1.999999999999971800 ) ) ;
#17234=CARTESIAN_POINT ( 'NONE',  ( 14.00000000000006750, 2.000000000000112799, 0.000000000000000000 ) ) ;
#17267=CARTESIAN_POINT ( 'NONE',  ( 0.000000000000000000, 0.000000000000000000, 0.000000000000000000 ) ) ;
#17287=ADVANCED_FACE ( 'NONE', ( #18018 ), #20805, .T. ) ;
#17301=CARTESIAN_POINT ( 'NONE',  ( 15.62500000000013856, -1.414213562372979016, -1.414213562373145550 ) ) ;
#17305=CARTESIAN_POINT ( 'NONE',  ( 14.12499999999999822, 5.551115123125782702E-14, -2.649519052838444910 ) ) ;
#17325=CARTESIAN_POINT ( 'NONE',  ( 22.18750000000018119, 0.8284271247464156662, 1.999999999999971800 ) ) ;
#17337=CARTESIAN_POINT ( 'NONE',  ( 18.68750000000005329, -1.097466725451499370, 2.649519052838238409 ) ) ;
#17345=EDGE_CURVE ( 'NONE', #26264, #25850, #23928, .T. ) ;
#17375=ORIENTED_EDGE ( 'NONE', *, *, #6987, .F. ) ;
#17382=CARTESIAN_POINT ( 'NONE',  ( 15.25000000000012434, 1.110223024625156540E-13, 1.999999999999946265 ) ) ;
#17398=CARTESIAN_POINT ( 'NONE',  ( 13.14882486540533257, -2.499999999999844569, 1.035533905932689347 ) ) ;
#17402=( BOUNDED_CURVE ( )  B_SPLINE_CURVE ( 2, ( #15278, #24605, #19568, #13143, #17581, #1417, #23056, #8486, #19857 ),
 .UNSPECIFIED., .F., .T. ) 
 B_SPLINE_CURVE_WITH_KNOTS ( ( 3, 2, 2, 2, 3 ),
 ( 0.01562500000000000000, 0.02343750000000000000, 0.03125000000000000000, 0.03906250000000000000, 0.04687500000000000000 ),
 .UNSPECIFIED. ) 
 CURVE ( )  GEOMETRIC_REPRESENTATION_ITEM ( )  RATIONAL_B_SPLINE_CURVE ( ( 1.000000000000000000, 0.9238795325112867385, 1.000000000000000000, 0.9238795325112867385, 1.000000000000000000, 0.9238795325112867385, 1.000000000000000000, 0.9238795325112867385, 1.000000000000000000 ) ) 
 REPRESENTATION_ITEM ( '' )  );
#17406=( LENGTH_UNIT ( ) NAMED_UNIT ( * ) SI_UNIT ( .MILLI., .METRE. ) );
#17409=CARTESIAN_POINT ( 'NONE',  ( 20.77382486540531303, 2.500000000000144773, 1.035533905932689347 ) ) ;
#17414=CARTESIAN_POINT ( 'NONE',  ( 25.00000000000015987, -1.873492889144789952, -1.873492889145123019 ) ) ;
#17416=CARTESIAN_POINT ( 'NONE',  ( 18.60117513459491434, -1.035533905932749299, 2.499999999999964473 ) ) ;
#17419=LINE ( 'NONE', #1242, #3749 ) ;
#17437=CARTESIAN_POINT ( 'NONE',  ( 14.18749999999996270, 0.8284271247462955401, 2.000000000000031530 ) ) ;
#17447=CARTESIAN_POINT ( 'NONE',  ( 16.93750000000001421, 2.000000000000151879, -0.8284271247462354770 ) ) ;
#17471=CARTESIAN_POINT ( 'NONE',  ( 21.50000000000004619, -1.999999999999890754, -1.665334536937734811E-13 ) ) ;
#17472=CARTESIAN_POINT ( 'NONE',  ( 10.58632486540522777, 1.767766952966487448, -1.767766952966487448 ) ) ;
#17481=CARTESIAN_POINT ( 'NONE',  ( 24.88665106358411094, 0.9137963255674127483, -1.910487928109039002 ) ) ;
#17503=CARTESIAN_POINT ( 'NONE',  ( 24.00000000000013145, 2.000000000000057288, -1.665334536937734811E-13 ) ) ;
#17512=CARTESIAN_POINT ( 'NONE',  ( 15.25000000000012434, -1.873492889144789952, -1.873492889145123019 ) ) ;
#17521=COLOUR_RGB ( '', 0.66274510, 0.83137255, 0.94901961) ;
#17522=CARTESIAN_POINT ( 'NONE',  ( 24.95539562619975271, 2.044604373800484876, -0.2498804828010667833 ) ) ;
#17535=CARTESIAN_POINT ( 'NONE',  ( 14.31250000000002132, -0.8284271247461152399, 2.000000000000151879 ) ) ;
#17536=CARTESIAN_POINT ( 'NONE',  ( -2.081668171172168020E-16, -5.204170427930420051E-17, 2.499999999999999112 ) ) ;
#17539=CARTESIAN_POINT ( 'NONE',  ( 13.78867513459489125, -2.499999999999780176, -1.110223024625156540E-13 ) ) ;
#17551=CARTESIAN_POINT ( 'NONE',  ( 17.53867513459494987, 1.665334536937734811E-13, 2.499999999999946709 ) ) ;
#17581=CARTESIAN_POINT ( 'NONE',  ( 10.28867513459494276, 2.500000000000057732, -1.665334536937734811E-13 ) ) ;
#17591=CARTESIAN_POINT ( 'NONE',  ( 13.93750000000017941, 2.000000000000151879, -0.8284271247462354770 ) ) ;
#17592=ADVANCED_FACE ( 'NONE', ( #3912 ), #11024, .T. ) ;
#17602=CARTESIAN_POINT ( 'NONE',  ( 16.18750000000014566, 0.8284271247462955401, 2.000000000000031530 ) ) ;
#17606=CARTESIAN_POINT ( 'NONE',  ( 15.00000000000015277, -1.873492889144845464, -1.873492889145011997 ) ) ;
#17610=LINE ( 'NONE', #10532, #29726 ) ;
#17621=DIRECTION ( 'NONE',  ( -1.000000000000000000, -1.665334536937731113E-16, 1.526556658859586792E-16 ) ) ;
#17640=ORIENTED_EDGE ( 'NONE', *, *, #18921, .T. ) ;
#17651=CARTESIAN_POINT ( 'NONE',  ( 10.14882486540516204, -2.499999999999964473, 1.035533905932869425 ) ) ;
#17661=CARTESIAN_POINT ( 'NONE',  ( 14.56250000000001954, 2.649519052838419153, -1.097466725451499370 ) ) ;
#17703=CARTESIAN_POINT ( 'NONE',  ( 23.56250000000001066, 2.649519052838298805, -1.097466725451559322 ) ) ;
#17710=CARTESIAN_POINT ( 'NONE',  ( 10.72617513459493388, -2.499999999999844569, 1.035533905932809473 ) ) ;
#17711=CARTESIAN_POINT ( 'NONE',  ( 11.31250000000006395, -0.8284271247460552878, 2.000000000000031530 ) ) ;
#17720=CARTESIAN_POINT ( 'NONE',  ( 24.43750000000014921, 2.649519052838478661, 1.097466725451499370 ) ) ;
#17746=CARTESIAN_POINT ( 'NONE',  ( 14.93750000000010303, 2.000000000000151879, -0.8284271247462955401 ) ) ;
#17755=CARTESIAN_POINT ( 'NONE',  ( 17.18750000000013500, 0.8284271247463557142, 1.999999999999971800 ) ) ;
#17756=ORIENTED_EDGE ( 'NONE', *, *, #24115, .T. ) ;
#17760=CARTESIAN_POINT ( 'NONE',  ( 14.18750000000002487, 1.097466725451559322, -2.649519052838298805 ) ) ;
#17780=ADVANCED_FACE ( 'NONE', ( #20683, #16414 ), #4377, .F. ) ;
#17795=ORIENTED_EDGE ( 'NONE', *, *, #8367, .F. ) ;
#17797=CARTESIAN_POINT ( 'NONE',  ( 16.37500000000008527, 2.649519052838500421, 0.000000000000000000 ) ) ;
#17813=CARTESIAN_POINT ( 'NONE',  ( 10.04463841219782694, -1.279379774532318326, 2.256154131400250673 ) ) ;
#17823=CARTESIAN_POINT ( 'NONE',  ( 15.12500000000005507, -2.649519052838222866, 0.000000000000000000 ) ) ;
#17833=EDGE_LOOP ( 'NONE', ( #456, #28692 ) ) ;
#17836=VERTEX_POINT ( 'NONE', #6994 ) ;
#17847=ORIENTED_EDGE ( 'NONE', *, *, #5092, .T. ) ;
#17848=CARTESIAN_POINT ( 'NONE',  ( 10.81250000000001243, 0.8284271247461753029, -2.000000000000091926 ) ) ;
#17849=LINE ( 'NONE', #17536, #16725 ) ;
#17850=EDGE_CURVE ( 'NONE', #25850, #3562, #11211, .T. ) ;
#17895=DIRECTION ( 'NONE',  ( -1.000000000000000000, -1.665334536937731113E-16, 1.526556658859586792E-16 ) ) ;
#17899=SURFACE_STYLE_FILL_AREA ( #8331 ) ;
#17904=CARTESIAN_POINT ( 'NONE',  ( 14.62500000000008171, -1.414213562372979016, -1.414213562373145550 ) ) ;
#17915=CARTESIAN_POINT ( 'NONE',  ( 18.87500000000008527, 1.414213562373256572, -1.414213562373090038 ) ) ;
#17927=CARTESIAN_POINT ( 'NONE',  ( 17.64882486540520645, 2.500000000000144773, -1.035533905932929599 ) ) ;
#17965=CARTESIAN_POINT ( 'NONE',  ( 10.21132486540524198, -2.499999999999835687, -1.110223024625156540E-13 ) ) ;
#17973=CARTESIAN_POINT ( 'NONE',  ( 16.37500000000016698, 1.110223024625156540E-13, -2.649519052838389399 ) ) ;
#18000=CARTESIAN_POINT ( 'NONE',  ( 13.56250000000003375, -1.999999999999971800, -0.8284271247462354770 ) ) ;
#18014=CARTESIAN_POINT ( 'NONE',  ( 0.000000000000000000, 0.000000000000000000, 0.000000000000000000 ) ) ;
#18018=FACE_OUTER_BOUND ( 'NONE', #10610, .T. ) ;
#18023=CARTESIAN_POINT ( 'NONE',  ( 10.78867513459497118, -2.499999999999946709, -5.551115123125782702E-14 ) ) ;
#18024=CARTESIAN_POINT ( 'NONE',  ( 9.625000000000133227, -1.414213562372979016, -1.414213562373145550 ) ) ;
#18029=CARTESIAN_POINT ( 'NONE',  ( 0.000000000000000000, 0.000000000000000000, 0.000000000000000000 ) ) ;
#18031=CARTESIAN_POINT ( 'NONE',  ( 21.83632486540532014, 1.767766952966487448, 1.767766952966376426 ) ) ;
#18036=CARTESIAN_POINT ( 'NONE',  ( 21.75000000000007461, 2.220446049250313081E-13, -2.000000000000001776 ) ) ;
#18051=FILL_AREA_STYLE ('',( #8649 ) ) ;
#18066=CARTESIAN_POINT ( 'NONE',  ( 12.87500000000008171, 1.414213562373312083, -1.414213562373034527 ) ) ;
#18079=EDGE_CURVE ( 'NONE', #3562, #4040, #22217, .T. ) ;
#18090=EDGE_CURVE ( 'NONE', #16041, #5962, #27484, .T. ) ;
#18098=LINE ( 'NONE', #5922, #3280 ) ;
#18117=CARTESIAN_POINT ( 'NONE',  ( 13.12500000000010836, -2.649519052838000821, -5.551115123125782702E-14 ) ) ;
#18123=EDGE_LOOP ( 'NONE', ( #18919, #29928, #5025, #736 ) ) ;
#18145=CARTESIAN_POINT ( 'NONE',  ( 5.000000000000088818, 5.637083940101657433E-14, -6.000000000000056843 ) ) ;
#18172=FACE_OUTER_BOUND ( 'NONE', #25373, .T. ) ;
#18181=CARTESIAN_POINT ( 'NONE',  ( 24.00000000000013145, 2.000000000000057288, -1.665334536937734811E-13 ) ) ;
#18188=CARTESIAN_POINT ( 'NONE',  ( 12.16367513459487526, 1.767766952966487448, -1.767766952966320915 ) ) ;
#18198=SURFACE_SIDE_STYLE ('',( #25067 ) ) ;
#18200=EDGE_LOOP ( 'NONE', ( #15280, #14761, #7142, #2312 ) ) ;
#18203=CARTESIAN_POINT ( 'NONE',  ( 13.25000000000017764, 5.551115123125782702E-14, 1.999999999999890754 ) ) ;
#18209=( BOUNDED_CURVE ( )  B_SPLINE_CURVE ( 2, ( #100, #28041, #7164, #16128, #16579, #18412, #1952, #30359, #25604 ),
 .UNSPECIFIED., .F., .T. ) 
 B_SPLINE_CURVE_WITH_KNOTS ( ( 3, 2, 2, 2, 3 ),
 ( 0.8281250000000000000, 0.8359375000000000000, 0.8437500000000000000, 0.8515625000000000000, 0.8593750000000000000 ),
 .UNSPECIFIED. ) 
 CURVE ( )  GEOMETRIC_REPRESENTATION_ITEM ( )  RATIONAL_B_SPLINE_CURVE ( ( 1.000000000000000000, 0.9238795325112867385, 1.000000000000000000, 0.9238795325112867385, 1.000000000000000000, 0.9238795325112867385, 1.000000000000000000, 0.9238795325112867385, 1.000000000000000000 ) ) 
 REPRESENTATION_ITEM ( '' )  );
#18211=CARTESIAN_POINT ( 'NONE',  ( 12.56250000000007638, -1.999999999999851674, -0.8284271247462354770 ) ) ;
#18214=CARTESIAN_POINT ( 'NONE',  ( 18.58632486540534501, 1.767766952966431937, -1.767766952966431937 ) ) ;
#18215=CARTESIAN_POINT ( 'NONE',  ( 10.37500000000005151, -1.414213562373034527, 1.414213562372756972 ) ) ;
#18224=DIRECTION ( 'NONE',  ( -8.326672684688675286E-17, -2.081668171172168821E-17, 1.000000000000000000 ) ) ;
#18233=CARTESIAN_POINT ( 'NONE',  ( 21.00000000000007461, 2.000000000000057288, 0.000000000000000000 ) ) ;
#18239=FILL_AREA_STYLE ('',( #28021 ) ) ;
#18259=DIRECTION ( 'NONE',  ( 1.000000000000000000, 0.000000000000000000, 0.000000000000000000 ) ) ;
#18274=CARTESIAN_POINT ( 'NONE',  ( 12.58632486540531303, 1.767766952966487448, -1.767766952966487448 ) ) ;
#18298=CARTESIAN_POINT ( 'NONE',  ( 11.81250000000006040, 0.8284271247463557142, -2.000000000000031530 ) ) ;
#18316=CARTESIAN_POINT ( 'NONE',  ( 20.06250000000002842, -2.649519052838238409, 1.097466725451559322 ) ) ;
#18336=CARTESIAN_POINT ( 'NONE',  ( 23.62500000000000711, -1.414213562372923505, -1.414213562373145550 ) ) ;
#18345=CARTESIAN_POINT ( 'NONE',  ( 12.47617513459493921, 1.035533905932869425, 2.499999999999844569 ) ) ;
#18361=CARTESIAN_POINT ( 'NONE',  ( 14.33632486540525974, -1.767766952966376426, -1.767766952966320915 ) ) ;
#18366=CARTESIAN_POINT ( 'NONE',  ( 14.50000000000012434, -1.999999999999779732, -5.551115123125782702E-14 ) ) ;
#18388=CARTESIAN_POINT ( 'NONE',  ( 18.43749999999999289, -1.999999999999971800, 0.8284271247462354770 ) ) ;
#18389=DIRECTION ( 'NONE',  ( -1.000000000000000000, -1.665334536937731113E-16, 1.526556658859586792E-16 ) ) ;
#18398=CARTESIAN_POINT ( 'NONE',  ( 11.58632486540531126, 1.767766952966487448, -1.767766952966431937 ) ) ;
#18412=CARTESIAN_POINT ( 'NONE',  ( 23.35117513459490368, 2.500000000000084821, 1.035533905932749299 ) ) ;
#18439=CARTESIAN_POINT ( 'NONE',  ( 23.06250000000007816, -1.097466725451379244, -2.649519052838358757 ) ) ;
#18451=CARTESIAN_POINT ( 'NONE',  ( 23.14882486540521711, -2.499999999999964473, 1.035533905932749299 ) ) ;
#18462=CARTESIAN_POINT ( 'NONE',  ( 22.00000000000015987, -1.873492889144789952, 1.873492889144900975 ) ) ;
#18470=CARTESIAN_POINT ( 'NONE',  ( 17.08632486540531659, -1.767766952966209892, 1.767766952966431937 ) ) ;
#18484=CARTESIAN_POINT ( 'NONE',  ( 23.00000000000013145, 2.000000000000168310, 0.000000000000000000 ) ) ;
#18516=CARTESIAN_POINT ( 'NONE',  ( 12.62500000000013678, -1.414213562372979016, -1.414213562373145550 ) ) ;
#18525=CARTESIAN_POINT ( 'NONE',  ( 2.081668171172167281E-16, 3.582034040661430693E-16, -2.499999999999999112 ) ) ;
#18539=CARTESIAN_POINT ( 'NONE',  ( 20.56250000000014566, -1.999999999999911626, -0.8284271247462354770 ) ) ;
#18540=CARTESIAN_POINT ( 'NONE',  ( -2.081668171172168020E-16, -5.204170427930420051E-17, 2.499999999999999112 ) ) ;
#18573=( BOUNDED_CURVE ( )  B_SPLINE_CURVE ( 2, ( #10568, #24372, #17195, #20082, #12742, #29426, #29116, #10889, #22386 ),
 .UNSPECIFIED., .F., .T. ) 
 B_SPLINE_CURVE_WITH_KNOTS ( ( 3, 2, 2, 2, 3 ),
 ( 0.7031250000000000000, 0.7109375000000000000, 0.7187500000000000000, 0.7265625000000000000, 0.7343750000000000000 ),
 .UNSPECIFIED. ) 
 CURVE ( )  GEOMETRIC_REPRESENTATION_ITEM ( )  RATIONAL_B_SPLINE_CURVE ( ( 1.000000000000000000, 0.9238795325112867385, 1.000000000000000000, 0.9238795325112867385, 1.000000000000000000, 0.9238795325112867385, 1.000000000000000000, 0.9238795325112867385, 1.000000000000000000 ) ) 
 REPRESENTATION_ITEM ( '' )  );
#18577=CARTESIAN_POINT ( 'NONE',  ( 9.874999999999994671, 1.110223024625156540E-13, 2.649519052838167354 ) ) ;
#18588=CARTESIAN_POINT ( 'NONE',  ( 21.06250000000013500, -1.097466725451439196, -2.649519052838419153 ) ) ;
#18596=CARTESIAN_POINT ( 'NONE',  ( 10.62500000000013500, -1.414213562372979016, -1.414213562373090038 ) ) ;
#18612=VERTEX_POINT ( 'NONE', #16619 ) ;
#18613=CARTESIAN_POINT ( 'NONE',  ( 21.56250000000010303, 2.649519052838419153, -1.097466725451559322 ) ) ;
#18622=DIRECTION ( 'NONE',  ( -1.000000000000000000, -1.665334536937731113E-16, 1.526556658859586792E-16 ) ) ;
#18629=CARTESIAN_POINT ( 'NONE',  ( 10.68750000000007283, -1.097466725451499370, 2.649519052838178457 ) ) ;
#18632=CARTESIAN_POINT ( 'NONE',  ( 21.43750000000007105, -1.999999999999911626, 0.8284271247461753029 ) ) ;
#18640=CARTESIAN_POINT ( 'NONE',  ( 24.62490920072287892, -2.016120031034378091, 1.292072678355042914 ) ) ;
#18641=LINE ( 'NONE', #20632, #12617 ) ;
#18651=ORIENTED_EDGE ( 'NONE', *, *, #5092, .F. ) ;
#18665=ORIENTED_EDGE ( 'NONE', *, *, #14682, .T. ) ;
#18666=CARTESIAN_POINT ( 'NONE',  ( 11.25000000000001066, 1.110223024625156540E-13, 1.999999999999946265 ) ) ;
#18679=CARTESIAN_POINT ( 'NONE',  ( 19.35117513459490013, 2.500000000000084821, 1.035533905932629173 ) ) ;
#18691=CARTESIAN_POINT ( 'NONE',  ( 19.62500000000008527, -1.414213562372979016, -1.414213562373145550 ) ) ;
#18728=CARTESIAN_POINT ( 'NONE',  ( 11.56250000000000000, 2.649519052838298805, -1.097466725451559322 ) ) ;
#18746=CARTESIAN_POINT ( 'NONE',  ( 22.81250000000005329, -2.649519052838178457, 1.097466725451559322 ) ) ;
#18767=CARTESIAN_POINT ( 'NONE',  ( 22.68750000000008882, 2.649519052838538613, 1.097466725451499370 ) ) ;
#18772=ORIENTED_EDGE ( 'NONE', *, *, #13583, .T. ) ;
#18777=CARTESIAN_POINT ( 'NONE',  ( 22.02382486540538764, -1.035533905932629173, 2.499999999999904521 ) ) ;
#18780=EDGE_LOOP ( 'NONE', ( #5119, #16300, #22115, #19187 ) ) ;
#18789=CARTESIAN_POINT ( 'NONE',  ( 17.93750000000012434, 2.000000000000091926, -0.8284271247463557142 ) ) ;
#18805=AXIS2_PLACEMENT_3D ( 'NONE', #20700, #11038, #18259 ) ;
#18807=ORIENTED_EDGE ( 'NONE', *, *, #7772, .F. ) ;
#18842=CARTESIAN_POINT ( 'NONE',  ( 16.68750000000013856, -0.8284271247461753029, -2.000000000000151879 ) ) ;
#18850=DIRECTION ( 'NONE',  ( -1.000000000000000000, -1.665334536937731113E-16, -8.326672684688674053E-17 ) ) ;
#18856=CARTESIAN_POINT ( 'NONE',  ( 21.37500000000011724, -1.414213562373090038, 1.414213562373034527 ) ) ;
#18875=CARTESIAN_POINT ( 'NONE',  ( 24.48000116661930292, 0.3094390903118284797, -2.499999999999972911 ) ) ;
#18879=CARTESIAN_POINT ( 'NONE',  ( 24.25000000000018829, 1.110223024625156540E-13, 2.000000000000001776 ) ) ;
#18888=DIRECTION ( 'NONE',  ( -1.000000000000000000, -1.665334536937731113E-16, 1.526556658859586792E-16 ) ) ;
#18896=VERTEX_POINT ( 'NONE', #15118 ) ;
#18900=CARTESIAN_POINT ( 'NONE',  ( 23.56250000000009948, 1.097466725451679892, 2.649519052838298805 ) ) ;
#18907=DIRECTION ( 'NONE',  ( -1.000000000000000000, -1.665334536937731113E-16, 1.526556658859586792E-16 ) ) ;
#18919=ORIENTED_EDGE ( 'NONE', *, *, #9514, .F. ) ;
#18920=CARTESIAN_POINT ( 'NONE',  ( 22.81250000000002132, 1.097466725451559322, 2.649519052838298805 ) ) ;
#18921=EDGE_CURVE ( 'NONE', #17836, #27181, #20423, .T. ) ;
#18944=CARTESIAN_POINT ( 'NONE',  ( 9.937500000000024869, -2.649519052838178457, -1.097466725451559322 ) ) ;
#18946=CARTESIAN_POINT ( 'NONE',  ( 20.31250000000012079, -0.8284271247461152399, 2.000000000000031530 ) ) ;
#18950=CARTESIAN_POINT ( 'NONE',  ( 15.03867513459491967, 1.665334536937734811E-13, -2.500000000000057732 ) ) ;
#18955=DIRECTION ( 'NONE',  ( -1.000000000000000000, -1.665334536937731113E-16, 1.526556658859586792E-16 ) ) ;
#18956=CARTESIAN_POINT ( 'NONE',  ( 14.41367513459493388, 1.767766952966431937, 1.767766952966376426 ) ) ;
#18967=CARTESIAN_POINT ( 'NONE',  ( 12.31250000000004974, -0.8284271247461753029, 2.000000000000091926 ) ) ;
#18987=CARTESIAN_POINT ( 'NONE',  ( 18.46132486540535922, 1.665334536937734811E-13, -2.500000000000113243 ) ) ;
#19007=CARTESIAN_POINT ( 'NONE',  ( 19.87500000000017053, 1.414213562373312083, -1.414213562373145550 ) ) ;
#19011=ORIENTED_EDGE ( 'NONE', *, *, #22293, .F. ) ;
#19035=CARTESIAN_POINT ( 'NONE',  ( 23.00000000000013145, 2.000000000000168310, 0.000000000000000000 ) ) ;
#19049=CARTESIAN_POINT ( 'NONE',  ( 18.56250000000008171, 1.097466725451679892, 2.649519052838358757 ) ) ;
#19071=EDGE_LOOP ( 'NONE', ( #8553, #27876, #6957, #7706 ) ) ;
#19072=CARTESIAN_POINT ( 'NONE',  ( 18.81250000000001776, 1.097466725451559322, 2.649519052838419153 ) ) ;
#19086=CARTESIAN_POINT ( 'NONE',  ( 11.75000000000012079, -1.873492889144845464, 1.873492889144900975 ) ) ;
#19089=CARTESIAN_POINT ( 'NONE',  ( 17.62500000000008527, -1.414213562372923505, -1.414213562373145550 ) ) ;
#19097=CARTESIAN_POINT ( 'NONE',  ( 15.46132486540530238, 1.110223024625156540E-13, -2.500000000000057732 ) ) ;
#19098=CARTESIAN_POINT ( 'NONE',  ( 14.28867513459491967, 2.500000000000224265, -5.551115123125782702E-14 ) ) ;
#19113=EDGE_CURVE ( 'NONE', #23217, #29417, #21882, .T. ) ;
#19116=ADVANCED_FACE ( 'NONE', ( #8960 ), #13596, .T. ) ;
#19132=DIRECTION ( 'NONE',  ( -1.000000000000000000, -1.665334536937731113E-16, 1.526556658859586792E-16 ) ) ;
#19133=CYLINDRICAL_SURFACE ( 'NONE', #23439, 2.499999999999999112 ) ;
#19144=CARTESIAN_POINT ( 'NONE',  ( 22.75000000000015987, 1.110223024625156540E-13, -2.000000000000168310 ) ) ;
#19148=CARTESIAN_POINT ( 'NONE',  ( 16.00000000000012434, -1.873492889144789952, -1.873492889145067508 ) ) ;
#19149=ADVANCED_FACE ( 'NONE', ( #12988 ), #1727, .T. ) ;
#19169=CARTESIAN_POINT ( 'NONE',  ( 24.56250000000017764, -1.999999999999911626, -0.8284271247462354770 ) ) ;
#19171=CARTESIAN_POINT ( 'NONE',  ( 24.50000000000010658, 5.551115123125782702E-14, -5.551115123125782702E-14 ) ) ;
#19178=EDGE_CURVE ( 'NONE', #28765, #21961, #7668, .T. ) ;
#19187=ORIENTED_EDGE ( 'NONE', *, *, #8021, .T. ) ;
#19206=CARTESIAN_POINT ( 'NONE',  ( 18.02382486540526330, -1.035533905932629173, 2.499999999999904521 ) ) ;
#19216=CARTESIAN_POINT ( 'NONE',  ( 22.47617513459494631, 1.035533905932869425, 2.499999999999904521 ) ) ;
#19225=CARTESIAN_POINT ( 'NONE',  ( 24.08632486540529527, -1.767766952966265404, 1.767766952966376426 ) ) ;
#19227=CARTESIAN_POINT ( 'NONE',  ( 11.50000000000012079, 1.873492889145067508, 1.873492889144734441 ) ) ;
#19230=CARTESIAN_POINT ( 'NONE',  ( 18.68750000000005329, -0.8284271247461753029, -1.999999999999971800 ) ) ;
#19234=AXIS2_PLACEMENT_3D ( 'NONE', #16031, #4143, #13723 ) ;
#19235=CARTESIAN_POINT ( 'NONE',  ( 12.39882486540519047, -1.035533905932629173, -2.500000000000024425 ) ) ;
#19243=CARTESIAN_POINT ( 'NONE',  ( 0.000000000000000000, 0.000000000000000000, 0.000000000000000000 ) ) ;
#19251=CARTESIAN_POINT ( 'NONE',  ( 11.75000000000012079, 1.665334536937734811E-13, -2.000000000000057288 ) ) ;
#19252=EDGE_CURVE ( 'NONE', #23786, #8065, #9844, .T. ) ;
#19263=CARTESIAN_POINT ( 'NONE',  ( 21.96132486540530593, 1.665334536937734811E-13, 2.499999999999946709 ) ) ;
#19278=CARTESIAN_POINT ( 'NONE',  ( 10.00000000000012257, -0.6095397824213422133, -2.424553825687569830 ) ) ;
#19296=CARTESIAN_POINT ( 'NONE',  ( 22.31250000000003197, -0.8284271247460553989, 2.000000000000031530 ) ) ;
#19306=CONICAL_SURFACE ( 'NONE', #6037, 2.499999999999999112, 0.7853981633974522758 ) ;
#19308=CARTESIAN_POINT ( 'NONE',  ( 17.03867513459494987, 1.665334536937734811E-13, -2.500000000000002220 ) ) ;
#19320=CARTESIAN_POINT ( 'NONE',  ( 9.250000000000092371, -1.873492889144789952, -1.873492889145123019 ) ) ;
#19326=ORIENTED_EDGE ( 'NONE', *, *, #27497, .F. ) ;
#19336=CARTESIAN_POINT ( 'NONE',  ( 19.37500000000017053, 2.649519052838444910, 0.000000000000000000 ) ) ;
#19357=CARTESIAN_POINT ( 'NONE',  ( 16.02382486540522777, -1.035533905932629173, 2.499999999999964473 ) ) ;
#19362=CIRCLE ( 'NONE', #6084, 1.999999999999998224 ) ;
#19366=CARTESIAN_POINT ( 'NONE',  ( 22.46132486540528106, 1.665334536937734811E-13, -2.500000000000113243 ) ) ;
#19368=CARTESIAN_POINT ( 'NONE',  ( 22.41367513459485750, 1.767766952966598470, 1.767766952966376426 ) ) ;
#19378=AXIS2_PLACEMENT_3D ( 'NONE', #8615, #11098, #10953 ) ;
#19380=CARTESIAN_POINT ( 'NONE',  ( 20.56250000000014566, -1.999999999999911626, -0.8284271247462354770 ) ) ;
#19419=ADVANCED_FACE ( 'NONE', ( #2163 ), #11873, .T. ) ;
#19437=CARTESIAN_POINT ( 'NONE',  ( 17.43750000000012790, -1.999999999999851674, 0.8284271247463557142 ) ) ;
#19444=CARTESIAN_POINT ( 'NONE',  ( 22.62500000000017408, -1.414213562372867994, -1.414213562373034527 ) ) ;
#19456=( LENGTH_UNIT ( ) NAMED_UNIT ( * ) SI_UNIT ( .MILLI., .METRE. ) );
#19467=CARTESIAN_POINT ( 'NONE',  ( 24.43750000000014921, -1.999999999999851674, 0.8284271247462354770 ) ) ;
#19477=ORIENTED_EDGE ( 'NONE', *, *, #13341, .T. ) ;
#19479=CARTESIAN_POINT ( 'NONE',  ( 19.68750000000009948, -1.097466725451499370, 2.649519052838238409 ) ) ;
#19499=CARTESIAN_POINT ( 'NONE',  ( 23.18750000000004974, 0.8284271247462955401, 1.999999999999851674 ) ) ;
#19505=ORIENTED_EDGE ( 'NONE', *, *, #2756, .F. ) ;
#19506=CARTESIAN_POINT ( 'NONE',  ( 16.87500000000011369, 1.110223024625156540E-13, 2.649519052838333888 ) ) ;
#19528=CARTESIAN_POINT ( 'NONE',  ( 14.18749999999996270, 0.8284271247462955401, 2.000000000000031530 ) ) ;
#19544=( BOUNDED_CURVE ( )  B_SPLINE_CURVE ( 2, ( #13616, #2217, #22962, #6667, #11620, #6345, #18214, #13775, #27685 ),
 .UNSPECIFIED., .F., .T. ) 
 B_SPLINE_CURVE_WITH_KNOTS ( ( 3, 2, 2, 2, 3 ),
 ( 0.3593750000000000000, 0.3671875000000000000, 0.3750000000000000000, 0.3828125000000000000, 0.3906250000000000000 ),
 .UNSPECIFIED. ) 
 CURVE ( )  GEOMETRIC_REPRESENTATION_ITEM ( )  RATIONAL_B_SPLINE_CURVE ( ( 1.000000000000000000, 0.9238795325112867385, 1.000000000000000000, 0.9238795325112867385, 1.000000000000000000, 0.9238795325112867385, 1.000000000000000000, 0.9238795325112867385, 1.000000000000000000 ) ) 
 REPRESENTATION_ITEM ( '' )  );
#19563=CARTESIAN_POINT ( 'NONE',  ( 24.84150635094622572, -1.291286745249641628E-13, -2.158493649053927044 ) ) ;
#19564=CARTESIAN_POINT ( 'NONE',  ( 11.46132486540535389, 1.110223024625156540E-13, -2.500000000000002220 ) ) ;
#19568=CARTESIAN_POINT ( 'NONE',  ( 10.16367513459492855, 1.767766952966431937, -1.767766952966431937 ) ) ;
#19587=CARTESIAN_POINT ( 'NONE',  ( 15.87500000000008349, 1.414213562373201061, -1.414213562373090038 ) ) ;
#19603=CYLINDRICAL_SURFACE ( 'NONE', #15428, 2.499999999999999112 ) ;
#19608=CARTESIAN_POINT ( 'NONE',  ( 10.71132486540515849, 2.500000000000168754, -5.551115123125782702E-14 ) ) ;
#19610=VERTEX_POINT ( 'NONE', #28386 ) ;
#19618=VERTEX_POINT ( 'NONE', #7795 ) ;
#19621=CARTESIAN_POINT ( 'NONE',  ( 20.12500000000003197, 5.551115123125782702E-14, -2.649519052838444910 ) ) ;
#19642=CARTESIAN_POINT ( 'NONE',  ( 24.37500000000014566, -1.414213562373034527, 1.414213562373034527 ) ) ;
#19648=CARTESIAN_POINT ( 'NONE',  ( 19.00000000000012790, -1.873492889144845464, 1.873492889144845464 ) ) ;
#19665=CARTESIAN_POINT ( 'NONE',  ( 20.08632486540521001, -1.767766952966265404, 1.767766952966376426 ) ) ;
#19668=CARTESIAN_POINT ( 'NONE',  ( 16.37500000000008527, -1.414213562373090038, 1.414213562373034527 ) ) ;
#19692=CARTESIAN_POINT ( 'NONE',  ( 10.68750000000004263, -0.8284271247460552878, -1.999999999999971800 ) ) ;
#19727=CARTESIAN_POINT ( 'NONE',  ( 17.56250000000009592, -1.999999999999851674, -0.8284271247461753029 ) ) ;
#19751=CARTESIAN_POINT ( 'NONE',  ( 21.75000000000007461, 2.220446049250313081E-13, -2.000000000000001776 ) ) ;
#19774=FACE_OUTER_BOUND ( 'NONE', #30001, .T. ) ;
#19787=CARTESIAN_POINT ( 'NONE',  ( 11.22617513459480598, 2.500000000000024425, -1.035533905932869425 ) ) ;
#19789=CARTESIAN_POINT ( 'NONE',  ( 15.87500000000000000, 1.665334536937734811E-13, 2.649519052838278377 ) ) ;
#19802=VERTEX_POINT ( 'NONE', #9494 ) ;
#19805=EDGE_LOOP ( 'NONE', ( #5215, #7418, #29875, #22265 ) ) ;
#19811=CARTESIAN_POINT ( 'NONE',  ( 16.06250000000006040, 2.000000000000151879, 0.8284271247461152399 ) ) ;
#19815=CARTESIAN_POINT ( 'NONE',  ( 13.53867513459486283, 1.110223024625156540E-13, 2.499999999999946709 ) ) ;
#19844=CARTESIAN_POINT ( 'NONE',  ( 25.00000000000013500, 2.000000000000279332, -5.551115123125782702E-14 ) ) ;
#19857=CARTESIAN_POINT ( 'NONE',  ( 10.53867513459491612, 5.551115123125782702E-14, 2.499999999999724665 ) ) ;
#19867=CARTESIAN_POINT ( 'NONE',  ( 15.56250000000003375, -1.999999999999851674, -0.8284271247462354770 ) ) ;
#19877=CARTESIAN_POINT ( 'NONE',  ( 15.18750000000007105, 0.8284271247462955401, 1.999999999999851674 ) ) ;
#19881=CARTESIAN_POINT ( 'NONE',  ( 13.93750000000005684, -2.649519052838238409, -1.097466725451559322 ) ) ;
#19895=MECHANICAL_DESIGN_GEOMETRIC_PRESENTATION_REPRESENTATION('',(#274),#16399);
#19906=CARTESIAN_POINT ( 'NONE',  ( 0.000000000000000000, 0.000000000000000000, 0.000000000000000000 ) ) ;
#19942=CARTESIAN_POINT ( 'NONE',  ( 13.43750000000012612, 1.097466725451619718, -2.649519052838298805 ) ) ;
#19963=CARTESIAN_POINT ( 'NONE',  ( 14.62500000000008171, -1.414213562372979016, -1.414213562373145550 ) ) ;
#19975=VECTOR ( 'NONE', #2058, 1000.000000000000000 ) ;
#19981=CARTESIAN_POINT ( 'NONE',  ( 24.56250000000011724, 2.649519052838358757, -1.097466725451559322 ) ) ;
#19997=CARTESIAN_POINT ( 'NONE',  ( 24.56250000000000000, 1.097466725451559322, 2.649519052838419153 ) ) ;
#20007=CARTESIAN_POINT ( 'NONE',  ( 22.46132486540528106, 1.665334536937734811E-13, -2.500000000000113243 ) ) ;
#20025=CARTESIAN_POINT ( 'NONE',  ( 15.25000000000012434, 1.110223024625156540E-13, 1.999999999999946265 ) ) ;
#20036=CARTESIAN_POINT ( 'NONE',  ( 18.62500000000003197, -1.414213562373034527, -1.414213562373090038 ) ) ;
#20040=CARTESIAN_POINT ( 'NONE',  ( 13.00000000000017764, -1.873492889144789952, -1.873492889145011997 ) ) ;
#20053=CARTESIAN_POINT ( 'NONE',  ( 24.99999999999999289, 5.587541955019290839E-14, -2.000000000000220268 ) ) ;
#20061=CARTESIAN_POINT ( 'NONE',  ( 10.52382486540521711, 1.035533905932929599, -2.499999999999904521 ) ) ;
#20070=CARTESIAN_POINT ( 'NONE',  ( 24.93195072464294171, 1.624501552917132496, -1.286961059548207498 ) ) ;
#20075=EDGE_LOOP ( 'NONE', ( #1536, #25257, #29813, #17640 ) ) ;
#20082=CARTESIAN_POINT ( 'NONE',  ( 21.22617513459490368, 2.500000000000144773, -1.035533905932929599 ) ) ;
#20086=AXIS2_PLACEMENT_3D ( 'NONE', #18014, #27331, #25028 ) ;
#20100=CARTESIAN_POINT ( 'NONE',  ( 14.43750000000014033, 1.097466725451739622, -2.649519052838358757 ) ) ;
#20128=CARTESIAN_POINT ( 'NONE',  ( 15.75000000000006928, 2.775557561562891351E-13, -2.000000000000057288 ) ) ;
#20143=CARTESIAN_POINT ( 'NONE',  ( 23.75000000000013145, 1.873492889145067508, 1.873492889144734441 ) ) ;
#20158=CARTESIAN_POINT ( 'NONE',  ( 21.58632486540529172, 1.767766952966598470, -1.767766952966487448 ) ) ;
#20188=CARTESIAN_POINT ( 'NONE',  ( 14.43750000000014033, -1.999999999999851674, 0.8284271247462955401 ) ) ;
#20200=CARTESIAN_POINT ( 'NONE',  ( 18.43749999999999645, -1.999999999999971800, 0.8284271247462354770 ) ) ;
#20211=PRODUCT_CONTEXT ( 'NONE', #8906, 'mechanical' ) ;
#20226=CARTESIAN_POINT ( 'NONE',  ( 22.56250000000011724, -1.999999999999851674, -0.8284271247462354770 ) ) ;
#20229=DIRECTION ( 'NONE',  ( -8.326672684688675286E-17, -2.081668171172168821E-17, 1.000000000000000000 ) ) ;
#20248=CARTESIAN_POINT ( 'NONE',  ( 0.000000000000000000, 0.000000000000000000, 0.000000000000000000 ) ) ;
#20254=CARTESIAN_POINT ( 'NONE',  ( 23.52382486540536277, 1.035533905932869425, -2.499999999999904521 ) ) ;
#20258=CARTESIAN_POINT ( 'NONE',  ( 11.47617513459495342, 1.035533905932869425, 2.499999999999844569 ) ) ;
#20261=CARTESIAN_POINT ( 'NONE',  ( 16.56250000000004974, 2.649519052838358757, -1.097466725451559322 ) ) ;
#20268=CARTESIAN_POINT ( 'NONE',  ( 20.96132486540536277, 5.551115123125782702E-14, 2.500000000000002220 ) ) ;
#20281=CARTESIAN_POINT ( 'NONE',  ( 13.43750000000012612, -1.999999999999971800, 0.8284271247462354770 ) ) ;
#20290=CARTESIAN_POINT ( 'NONE',  ( 24.52451905283846401, 1.480436431285038258E-13, 2.475480947161601275 ) ) ;
#20291=EDGE_CURVE ( 'NONE', #22378, #25453, #27862, .T. ) ;
#20294=FACE_OUTER_BOUND ( 'NONE', #28062, .T. ) ;
#20297=CARTESIAN_POINT ( 'NONE',  ( 24.31250000000006395, -1.097466725451379244, -2.649519052838419153 ) ) ;
#20304=CARTESIAN_POINT ( 'NONE',  ( 9.500000000000008882, -1.999999999999835243, 0.000000000000000000 ) ) ;
#20315=CARTESIAN_POINT ( 'NONE',  ( 24.06250000000009592, 2.000000000000091926, 0.8284271247461152399 ) ) ;
#20323=FACE_OUTER_BOUND ( 'NONE', #19805, .T. ) ;
#20327=ORIENTED_EDGE ( 'NONE', *, *, #835, .T. ) ;
#20336=CARTESIAN_POINT ( 'NONE',  ( 21.78867513459492500, -2.499999999999835687, -1.110223024625156540E-13 ) ) ;
#20341=CARTESIAN_POINT ( 'NONE',  ( 13.56250000000003197, -1.999999999999971800, -0.8284271247462354770 ) ) ;
#20345=CARTESIAN_POINT ( 'NONE',  ( 13.56250000000003375, 1.097466725451679892, 2.649519052838419153 ) ) ;
#20355=CARTESIAN_POINT ( 'NONE',  ( 17.71132486540530238, 2.500000000000057732, -1.665334536937734811E-13 ) ) ;
#20356=CARTESIAN_POINT ( 'NONE',  ( 19.52382486540523843, 1.035533905932869425, -2.499999999999964473 ) ) ;
#20363=CARTESIAN_POINT ( 'NONE',  ( 20.62500000000014211, -1.414213562372979016, -1.414213562373145550 ) ) ;
#20395=CARTESIAN_POINT ( 'NONE',  ( 13.81249999999996980, 1.097466725451619718, 2.649519052838358757 ) ) ;
#20420=ORIENTED_EDGE ( 'NONE', *, *, #28192, .F. ) ;
#20421=CARTESIAN_POINT ( 'NONE',  ( 11.12500000000010658, 1.414213562373201061, 1.414213562373034527 ) ) ;
#20423=( BOUNDED_CURVE ( )  B_SPLINE_CURVE ( 2, ( #19278, #26743, #2962 ),
 .UNSPECIFIED., .F., .T. ) 
 B_SPLINE_CURVE_WITH_KNOTS ( ( 3, 3 ),
 ( 0.01315883293251204553, 0.01562500000000000000 ),
 .UNSPECIFIED. ) 
 CURVE ( )  GEOMETRIC_REPRESENTATION_ITEM ( )  RATIONAL_B_SPLINE_CURVE ( ( 0.9671125746057327444, 0.9759710988694461076, 1.000000000000000000 ) ) 
 REPRESENTATION_ITEM ( '' )  );
#20444=CARTESIAN_POINT ( 'NONE',  ( 10.53867513459491612, 5.551115123125782702E-14, 2.499999999999724665 ) ) ;
#20448=DIRECTION ( 'NONE',  ( -1.000000000000000000, -1.665334536937731113E-16, 1.526556658859586792E-16 ) ) ;
#20457=CARTESIAN_POINT ( 'NONE',  ( 22.56250000000011724, -1.999999999999851674, -0.8284271247462354770 ) ) ;
#20465=DIRECTION ( 'NONE',  ( -8.326672684688675286E-17, -2.081668171172168821E-17, 1.000000000000000000 ) ) ;
#20480=CARTESIAN_POINT ( 'NONE',  ( 12.81250000000004441, 0.8284271247461753029, -2.000000000000091926 ) ) ;
#20490=CARTESIAN_POINT ( 'NONE',  ( 14.06250000000011546, 2.000000000000151879, 0.8284271247461753029 ) ) ;
#20493=CARTESIAN_POINT ( 'NONE',  ( 10.00000000000012079, -0.6095397824213422133, -2.424553825687569830 ) ) ;
#20495=CARTESIAN_POINT ( 'NONE',  ( 10.43750000000004796, -1.999999999999851674, 0.8284271247461753029 ) ) ;
#20516=CARTESIAN_POINT ( 'NONE',  ( 18.68750000000005329, -0.8284271247461753029, -1.999999999999971800 ) ) ;
#20526=CARTESIAN_POINT ( 'NONE',  ( 11.71132486540527040, 2.500000000000113243, -5.551115123125782702E-14 ) ) ;
#20528=ORIENTED_EDGE ( 'NONE', *, *, #28632, .F. ) ;
#20554=CARTESIAN_POINT ( 'NONE',  ( 12.87500000000010836, 5.551115123125782702E-14, 2.649519052838333888 ) ) ;
#20580=VERTEX_POINT ( 'NONE', #13371 ) ;
#20581=CARTESIAN_POINT ( 'NONE',  ( 12.87500000000008171, 1.414213562373312083, -1.414213562373034527 ) ) ;
#20596=CARTESIAN_POINT ( 'NONE',  ( 23.00000000000007461, -1.873492889144789952, 1.873492889144734441 ) ) ;
#20609=EDGE_CURVE ( 'NONE', #1806, #7693, #14959, .T. ) ;
#20610=CARTESIAN_POINT ( 'NONE',  ( 9.999999999999841904, 2.000000000000057288, -4.274358644806852681E-12 ) ) ;
#20621=CARTESIAN_POINT ( 'NONE',  ( 24.68750000000014566, -0.8284271247460552878, -2.000000000000151879 ) ) ;
#20622=FACE_OUTER_BOUND ( 'NONE', #23829, .T. ) ;
#20632=CARTESIAN_POINT ( 'NONE',  ( 2.081668171172167281E-16, 3.582034040661430693E-16, -2.499999999999999112 ) ) ;
#20637=DIRECTION ( 'NONE',  ( -8.326672684688675286E-17, -2.081668171172168821E-17, 1.000000000000000000 ) ) ;
#20638=ORIENTED_EDGE ( 'NONE', *, *, #1817, .F. ) ;
#20644=CARTESIAN_POINT ( 'NONE',  ( 13.96132486540527218, 1.110223024625156540E-13, 2.499999999999946709 ) ) ;
#20653=CARTESIAN_POINT ( 'NONE',  ( 13.06249999999998046, 2.000000000000151879, 0.8284271247461153509 ) ) ;
#20654=ORIENTED_EDGE ( 'NONE', *, *, #17345, .F. ) ;
#20678=LINE ( 'NONE', #23144, #13928 ) ;
#20683=FACE_BOUND ( 'NONE', #21886, .T. ) ;
#20700=CARTESIAN_POINT ( 'NONE',  ( 0.000000000000000000, 0.000000000000000000, 0.000000000000000000 ) ) ;
#20707=CARTESIAN_POINT ( 'NONE',  ( 21.46132486540527751, 5.551115123125782702E-14, -2.500000000000002220 ) ) ;
#20716=CARTESIAN_POINT ( 'NONE',  ( 10.00000000000014211, 1.983679448820493629, -0.6834733846401986890 ) ) ;
#20728=CARTESIAN_POINT ( 'NONE',  ( 22.68750000000008882, -1.097466725451439196, 2.649519052838358757 ) ) ;
#20735=CARTESIAN_POINT ( 'NONE',  ( 24.46132486540536632, 1.665334536937734811E-13, -2.500000000000002220 ) ) ;
#20738=CARTESIAN_POINT ( 'NONE',  ( 11.56250000000009059, -1.999999999999851674, -0.8284271247462354770 ) ) ;
#20758=CARTESIAN_POINT ( 'NONE',  ( 22.18750000000012434, -2.649519052838178457, -1.097466725451559322 ) ) ;
#20775=CARTESIAN_POINT ( 'NONE',  ( 18.91367513459496408, -1.767766952966265404, -1.767766952966376426 ) ) ;
#20778=CARTESIAN_POINT ( 'NONE',  ( 22.00000000000010303, 2.000000000000168310, 0.000000000000000000 ) ) ;
#20787=CARTESIAN_POINT ( 'NONE',  ( 24.52451905283846401, 1.480436431285038258E-13, 2.475480947161601275 ) ) ;
#20789=CARTESIAN_POINT ( 'NONE',  ( 13.46132486540532724, 1.665334536937734811E-13, -2.500000000000057732 ) ) ;
#20795=EDGE_LOOP ( 'NONE', ( #15250, #29752, #3368, #23115 ) ) ;
#20805=( BOUNDED_SURFACE ( )  B_SPLINE_SURFACE ( 1, 2, ( 
 ( #24883, #19981, #13112, #24576, #15244, #20297, #1537, #22292, #1221, #8290, #10632, #25030, #6299, #3835, #20143, #29333, #13262, #17703, #24737, #8609, #22450, #22603, #10945, #29643, #14181, #11715, #20596, #20909, #23218, #18920, #25803, #18767, #23518, #11411, #29945, #30255, #22902, #21058, #16331, #20758, #13563, #4753, #18462, #2459, #4452, #16628, #23370, #2314, #21211, #18613, #25948, #27783, #11875, #30407, #153, #9376, #1846, #6760, #28088, #16181, #9222, #16476, #11248, #2003, #27933, #30105, #8925, #6909, #25327, #7216, #9069, #9532, #7063, #18316, #25650, #28242, #27628, #13721, #23061, #4602, #16029, #6607, #25485, #13877, #14032, #2601, #14895, #887, #14606, #7655, #19648, #21661, #23807, #19072, #26538, #17063, #24236, #23958, #14751, #2741, #12020, #21357, #9828, #12463, #26242, #9982, #28681, #14327, #7797, #17210, #3045, #28987, #24096, #295, #28535, #10137, #7504, #5342, #9683, #28388, #12168, #751, #21514, #16775, #19506, #26098, #14472, #16917, #2896, #20261, #8730, #22407, #17973, #26679, #5788, #15204, #29443, #29136, #15680, #22564, #19789, #1494, #3336, #27286, #24988, #5950, #8418, #22712, #13074, #24537, #17512, #6259, #17823, #3938, #15372, #15524, #3486, #12763, #22105, #1182, #3794, #17661, #1344, #20100, #5642, #29607, #24694, #13368, #29753, #1654, #3637, #24845, #12916, #20395, #22253, #10906, #15045, #10591, #1042, #19942, #29291, #26984, #27143, #27897, #18117, #25444, #15984, #30062, #20554, #15838, #16294, #6871, #27585, #4712, #4256, #25137, #11679, #23332, #20866, #16139, #21022, #13833, #29905, #4102, #4567, #13676, #9032, #8885, #1802, #18728, #25614, #13524, #4408, #23178, #23484, #30370, #9338, #28051, #25283, #22864, #2122, #27435, #13993, #30217, #23017, #6563, #7023, #1963, #16441, #11525, #21172, #25766, #14145, #2422, #9181, #114, #18577, #11836, #24057, #12423, #5003, #7758, #3146, #17169, #3002, #26060, #19320, #9496, #16883 ),
 ( #28796, #4860, #710, #21317, #9790, #23769, #11987, #19169, #7469, #19467, #2857, #26202, #18879, #5448, #9642, #23916, #26492, #28352, #2563, #5153, #21622, #28201, #28642, #14568, #554, #9944, #260, #14857, #24201, #7613, #17023, #7176, #19035, #26351, #7327, #5301, #14714, #5906, #28947, #20226, #13191, #10719, #5750, #15486, #24953, #17325, #5601, #15005, #24345, #24811, #10398, #3761, #19751, #8211, #8056, #12876, #17471, #26786, #24496, #29249, #22983, #4674, #28014, #8999, #18233, #22674, #25410, #1617, #13638, #23143, #20363, #18539, #6686, #4532, #27865, #30337, #9147, #13798, #1767, #4062, #6986, #2242, #13957, #23298, #16406, #1924, #18691, #13486, #16107, #11330, #6527, #20989, #25576, #27402, #30029, #27551, #20833, #11644, #6367, #15949, #11169, #20516, #29869, #27704, #8850, #18388, #25248, #4221, #23446, #4971, #14539, #21136, #28608, #28467, #14679, #7578, #21736, #16991, #23879, #23591, #16556, #19437, #2968, #675, #10061, #28762, #23740, #7730, #4828, #16845, #9757, #26023, #9458, #18842, #2528, #11955, #9606, #21282, #220, #29212, #10362, #22494, #22333, #7879, #10513, #1267, #22179, #10678, #27070, #8336, #24615, #19867, #12691, #10216, #3260, #22024, #20025, #24459, #1113, #29372, #12838, #17746, #13155, #29541, #15290, #1427, #17904, #10836, #5419, #20188, #29066, #6035, #8031, #17437, #26750, #15128, #3412, #17591, #15453, #24174, #3117, #12539, #15611, #13449, #11294, #6799, #22797, #13302, #18203, #6656, #24924, #25377, #4190, #11132, #8819, #20480, #27521, #16223, #13605, #22950, #2057, #7548, #9573, #18967, #2641, #12060, #2787, #641, #9876, #482, #12215, #21555, #19251, #5235, #14647, #4643, #14076, #28135, #5682, #17711, #3379, #6000, #12805, #10024, #10327, #5534, #26876, #14940, #24278, #19692, #3225, #29035, #22146, #1089, #10484, #5838, #15253, #25037, #13413, #8465, #9503, #2430, #3992, #22760, #11842, #21179, #18024, #29649, #20304 ) ),
 .UNSPECIFIED., .F., .F., .T. ) 
 B_SPLINE_SURFACE_WITH_KNOTS ( ( 2, 2 ),
 ( 3, 2, 2, 2, 2, 2, 2, 2, 2, 2, 2, 2, 2, 2, 2, 2, 2, 2, 2, 2, 2, 2, 2, 2, 2, 2, 2, 2, 2, 2, 2, 2, 2, 2, 2, 2, 2, 2, 2, 2, 2, 2, 2, 2, 2, 2, 2, 2, 2, 2, 2, 2, 2, 2, 2, 2, 2, 2, 2, 2, 2, 2, 2, 2, 2, 2, 2, 2, 2, 2, 2, 2, 2, 2, 2, 2, 2, 2, 2, 2, 2, 2, 2, 2, 2, 2, 2, 2, 2, 2, 2, 2, 2, 2, 2, 2, 2, 2, 2, 2, 2, 2, 2, 2, 2, 2, 2, 2, 2, 2, 2, 2, 2, 2, 2, 2, 2, 2, 2, 2, 2, 2, 2, 2, 3 ),
 ( 0.000000000000000000, 1.000000000000000000 ),
 ( 0.000000000000000000, 0.007812500000000000000, 0.01562500000000000000, 0.02343750000000000000, 0.03125000000000000000, 0.03906250000000000000, 0.04687500000000000000, 0.05468750000000000000, 0.06250000000000000000, 0.07031250000000000000, 0.07812500000000000000, 0.08593750000000000000, 0.09375000000000000000, 0.1015625000000000000, 0.1093750000000000000, 0.1171875000000000000, 0.1250000000000000000, 0.1328125000000000000, 0.1406250000000000000, 0.1484375000000000000, 0.1562500000000000000, 0.1640625000000000000, 0.1718750000000000000, 0.1796875000000000000, 0.1875000000000000000, 0.1953125000000000000, 0.2031250000000000000, 0.2109375000000000000, 0.2187500000000000000, 0.2265625000000000000, 0.2343750000000000000, 0.2421875000000000000, 0.2500000000000000000, 0.2578125000000000000, 0.2656250000000000000, 0.2734375000000000000, 0.2812500000000000000, 0.2890625000000000000, 0.2968750000000000000, 0.3046875000000000000, 0.3125000000000000000, 0.3203125000000000000, 0.3281250000000000000, 0.3359375000000000000, 0.3437500000000000000, 0.3515625000000000000, 0.3593750000000000000, 0.3671875000000000000, 0.3750000000000000000, 0.3828125000000000000, 0.3906250000000000000, 0.3984375000000000000, 0.4062500000000000000, 0.4140625000000000000, 0.4218750000000000000, 0.4296875000000000000, 0.4375000000000000000, 0.4453125000000000000, 0.4531250000000000000, 0.4609375000000000000, 0.4687500000000000000, 0.4765625000000000000, 0.4843750000000000000, 0.4921875000000000000, 0.5000000000000000000, 0.5078125000000000000, 0.5156250000000000000, 0.5234375000000000000, 0.5312500000000000000, 0.5390625000000000000, 0.5468750000000000000, 0.5546875000000000000, 0.5625000000000000000, 0.5703125000000000000, 0.5781250000000000000, 0.5859375000000000000, 0.5937500000000000000, 0.6015625000000000000, 0.6093750000000000000, 0.6171875000000000000, 0.6250000000000000000, 0.6328125000000000000, 0.6406250000000000000, 0.6484375000000000000, 0.6562500000000000000, 0.6640625000000000000, 0.6718750000000000000, 0.6796875000000000000, 0.6875000000000000000, 0.6953125000000000000, 0.7031250000000000000, 0.7109375000000000000, 0.7187500000000000000, 0.7265625000000000000, 0.7343750000000000000, 0.7421875000000000000, 0.7500000000000000000, 0.7578125000000000000, 0.7656250000000000000, 0.7734375000000000000, 0.7812500000000000000, 0.7890625000000000000, 0.7968750000000000000, 0.8046875000000000000, 0.8125000000000000000, 0.8203125000000000000, 0.8281250000000000000, 0.8359375000000000000, 0.8437500000000000000, 0.8515625000000000000, 0.8593750000000000000, 0.8671875000000000000, 0.8750000000000000000, 0.8828125000000000000, 0.8906250000000000000, 0.8984375000000000000, 0.9062500000000000000, 0.9140625000000000000, 0.9218750000000000000, 0.9296875000000000000, 0.9375000000000000000, 0.9453125000000000000, 0.9531250000000000000, 0.9609375000000000000, 0.9687500000000000000 ),
 .UNSPECIFIED. ) 
 GEOMETRIC_REPRESENTATION_ITEM ( )  RATIONAL_B_SPLINE_SURFACE ( (
 ( 1.000000000000000000, 0.9238795325112867385, 1.000000000000000000, 0.9238795325112867385, 1.000000000000000000, 0.9238795325112867385, 1.000000000000000000, 0.9238795325112867385, 1.000000000000000000, 0.9238795325112867385, 1.000000000000000000, 0.9238795325112867385, 1.000000000000000000, 0.9238795325112867385, 1.000000000000000000, 0.9238795325112867385, 1.000000000000000000, 0.9238795325112867385, 1.000000000000000000, 0.9238795325112867385, 1.000000000000000000, 0.9238795325112867385, 1.000000000000000000, 0.9238795325112867385, 1.000000000000000000, 0.9238795325112867385, 1.000000000000000000, 0.9238795325112867385, 1.000000000000000000, 0.9238795325112867385, 1.000000000000000000, 0.9238795325112867385, 1.000000000000000000, 0.9238795325112867385, 1.000000000000000000, 0.9238795325112867385, 1.000000000000000000, 0.9238795325112867385, 1.000000000000000000, 0.9238795325112867385, 1.000000000000000000, 0.9238795325112867385, 1.000000000000000000, 0.9238795325112867385, 1.000000000000000000, 0.9238795325112867385, 1.000000000000000000, 0.9238795325112867385, 1.000000000000000000, 0.9238795325112867385, 1.000000000000000000, 0.9238795325112867385, 1.000000000000000000, 0.9238795325112867385, 1.000000000000000000, 0.9238795325112867385, 1.000000000000000000, 0.9238795325112867385, 1.000000000000000000, 0.9238795325112867385, 1.000000000000000000, 0.9238795325112867385, 1.000000000000000000, 0.9238795325112867385, 1.000000000000000000, 0.9238795325112867385, 1.000000000000000000, 0.9238795325112867385, 1.000000000000000000, 0.9238795325112867385, 1.000000000000000000, 0.9238795325112867385, 1.000000000000000000, 0.9238795325112867385, 1.000000000000000000, 0.9238795325112867385, 1.000000000000000000, 0.9238795325112867385, 1.000000000000000000, 0.9238795325112867385, 1.000000000000000000, 0.9238795325112867385, 1.000000000000000000, 0.9238795325112867385, 1.000000000000000000, 0.9238795325112867385, 1.000000000000000000, 0.9238795325112867385, 1.000000000000000000, 0.9238795325112867385, 1.000000000000000000, 0.9238795325112867385, 1.000000000000000000, 0.9238795325112867385, 1.000000000000000000, 0.9238795325112867385, 1.000000000000000000, 0.9238795325112867385, 1.000000000000000000, 0.9238795325112867385, 1.000000000000000000, 0.9238795325112867385, 1.000000000000000000, 0.9238795325112867385, 1.000000000000000000, 0.9238795325112867385, 1.000000000000000000, 0.9238795325112867385, 1.000000000000000000, 0.9238795325112867385, 1.000000000000000000, 0.9238795325112867385, 1.000000000000000000, 0.9238795325112867385, 1.000000000000000000, 0.9238795325112867385, 1.000000000000000000, 0.9238795325112867385, 1.000000000000000000, 0.9238795325112867385, 1.000000000000000000, 0.9238795325112867385, 1.000000000000000000, 0.9238795325112867385, 1.000000000000000000, 0.9238795325112867385, 1.000000000000000000, 0.9238795325112867385, 1.000000000000000000, 0.9238795325112867385, 1.000000000000000000, 0.9238795325112867385, 1.000000000000000000, 0.9238795325112867385, 1.000000000000000000, 0.9238795325112867385, 1.000000000000000000, 0.9238795325112867385, 1.000000000000000000, 0.9238795325112867385, 1.000000000000000000, 0.9238795325112867385, 1.000000000000000000, 0.9238795325112867385, 1.000000000000000000, 0.9238795325112867385, 1.000000000000000000, 0.9238795325112867385, 1.000000000000000000, 0.9238795325112867385, 1.000000000000000000, 0.9238795325112867385, 1.000000000000000000, 0.9238795325112867385, 1.000000000000000000, 0.9238795325112867385, 1.000000000000000000, 0.9238795325112867385, 1.000000000000000000, 0.9238795325112867385, 1.000000000000000000, 0.9238795325112867385, 1.000000000000000000, 0.9238795325112867385, 1.000000000000000000, 0.9238795325112867385, 1.000000000000000000, 0.9238795325112867385, 1.000000000000000000, 0.9238795325112867385, 1.000000000000000000, 0.9238795325112867385, 1.000000000000000000, 0.9238795325112867385, 1.000000000000000000, 0.9238795325112867385, 1.000000000000000000, 0.9238795325112867385, 1.000000000000000000, 0.9238795325112867385, 1.000000000000000000, 0.9238795325112867385, 1.000000000000000000, 0.9238795325112867385, 1.000000000000000000, 0.9238795325112867385, 1.000000000000000000, 0.9238795325112867385, 1.000000000000000000, 0.9238795325112867385, 1.000000000000000000, 0.9238795325112867385, 1.000000000000000000, 0.9238795325112867385, 1.000000000000000000, 0.9238795325112867385, 1.000000000000000000, 0.9238795325112867385, 1.000000000000000000, 0.9238795325112867385, 1.000000000000000000, 0.9238795325112867385, 1.000000000000000000, 0.9238795325112867385, 1.000000000000000000, 0.9238795325112867385, 1.000000000000000000, 0.9238795325112867385, 1.000000000000000000, 0.9238795325112867385, 1.000000000000000000, 0.9238795325112867385, 1.000000000000000000, 0.9238795325112867385, 1.000000000000000000, 0.9238795325112867385, 1.000000000000000000, 0.9238795325112867385, 1.000000000000000000, 0.9238795325112867385, 1.000000000000000000, 0.9238795325112867385, 1.000000000000000000, 0.9238795325112867385, 1.000000000000000000, 0.9238795325112867385, 1.000000000000000000, 0.9238795325112867385, 1.000000000000000000, 0.9238795325112867385, 1.000000000000000000, 0.9238795325112867385, 1.000000000000000000, 0.9238795325112867385, 1.000000000000000000, 0.9238795325112867385, 1.000000000000000000, 0.9238795325112867385, 1.000000000000000000, 0.9238795325112867385, 1.000000000000000000, 0.9238795325112867385, 1.000000000000000000, 0.9238795325112867385, 1.000000000000000000, 0.9238795325112867385, 1.000000000000000000, 0.9238795325112867385, 1.000000000000000000),
 ( 1.000000000000000000, 0.9238795325112867385, 1.000000000000000000, 0.9238795325112867385, 1.000000000000000000, 0.9238795325112867385, 1.000000000000000000, 0.9238795325112867385, 1.000000000000000000, 0.9238795325112867385, 1.000000000000000000, 0.9238795325112867385, 1.000000000000000000, 0.9238795325112867385, 1.000000000000000000, 0.9238795325112867385, 1.000000000000000000, 0.9238795325112867385, 1.000000000000000000, 0.9238795325112867385, 1.000000000000000000, 0.9238795325112867385, 1.000000000000000000, 0.9238795325112867385, 1.000000000000000000, 0.9238795325112867385, 1.000000000000000000, 0.9238795325112867385, 1.000000000000000000, 0.9238795325112867385, 1.000000000000000000, 0.9238795325112867385, 1.000000000000000000, 0.9238795325112867385, 1.000000000000000000, 0.9238795325112867385, 1.000000000000000000, 0.9238795325112867385, 1.000000000000000000, 0.9238795325112867385, 1.000000000000000000, 0.9238795325112867385, 1.000000000000000000, 0.9238795325112867385, 1.000000000000000000, 0.9238795325112867385, 1.000000000000000000, 0.9238795325112867385, 1.000000000000000000, 0.9238795325112867385, 1.000000000000000000, 0.9238795325112867385, 1.000000000000000000, 0.9238795325112867385, 1.000000000000000000, 0.9238795325112867385, 1.000000000000000000, 0.9238795325112867385, 1.000000000000000000, 0.9238795325112867385, 1.000000000000000000, 0.9238795325112867385, 1.000000000000000000, 0.9238795325112867385, 1.000000000000000000, 0.9238795325112867385, 1.000000000000000000, 0.9238795325112867385, 1.000000000000000000, 0.9238795325112867385, 1.000000000000000000, 0.9238795325112867385, 1.000000000000000000, 0.9238795325112867385, 1.000000000000000000, 0.9238795325112867385, 1.000000000000000000, 0.9238795325112867385, 1.000000000000000000, 0.9238795325112867385, 1.000000000000000000, 0.9238795325112867385, 1.000000000000000000, 0.9238795325112867385, 1.000000000000000000, 0.9238795325112867385, 1.000000000000000000, 0.9238795325112867385, 1.000000000000000000, 0.9238795325112867385, 1.000000000000000000, 0.9238795325112867385, 1.000000000000000000, 0.9238795325112867385, 1.000000000000000000, 0.9238795325112867385, 1.000000000000000000, 0.9238795325112867385, 1.000000000000000000, 0.9238795325112867385, 1.000000000000000000, 0.9238795325112867385, 1.000000000000000000, 0.9238795325112867385, 1.000000000000000000, 0.9238795325112867385, 1.000000000000000000, 0.9238795325112867385, 1.000000000000000000, 0.9238795325112867385, 1.000000000000000000, 0.9238795325112867385, 1.000000000000000000, 0.9238795325112867385, 1.000000000000000000, 0.9238795325112867385, 1.000000000000000000, 0.9238795325112867385, 1.000000000000000000, 0.9238795325112867385, 1.000000000000000000, 0.9238795325112867385, 1.000000000000000000, 0.9238795325112867385, 1.000000000000000000, 0.9238795325112867385, 1.000000000000000000, 0.9238795325112867385, 1.000000000000000000, 0.9238795325112867385, 1.000000000000000000, 0.9238795325112867385, 1.000000000000000000, 0.9238795325112867385, 1.000000000000000000, 0.9238795325112867385, 1.000000000000000000, 0.9238795325112867385, 1.000000000000000000, 0.9238795325112867385, 1.000000000000000000, 0.9238795325112867385, 1.000000000000000000, 0.9238795325112867385, 1.000000000000000000, 0.9238795325112867385, 1.000000000000000000, 0.9238795325112867385, 1.000000000000000000, 0.9238795325112867385, 1.000000000000000000, 0.9238795325112867385, 1.000000000000000000, 0.9238795325112867385, 1.000000000000000000, 0.9238795325112867385, 1.000000000000000000, 0.9238795325112867385, 1.000000000000000000, 0.9238795325112867385, 1.000000000000000000, 0.9238795325112867385, 1.000000000000000000, 0.9238795325112867385, 1.000000000000000000, 0.9238795325112867385, 1.000000000000000000, 0.9238795325112867385, 1.000000000000000000, 0.9238795325112867385, 1.000000000000000000, 0.9238795325112867385, 1.000000000000000000, 0.9238795325112867385, 1.000000000000000000, 0.9238795325112867385, 1.000000000000000000, 0.9238795325112867385, 1.000000000000000000, 0.9238795325112867385, 1.000000000000000000, 0.9238795325112867385, 1.000000000000000000, 0.9238795325112867385, 1.000000000000000000, 0.9238795325112867385, 1.000000000000000000, 0.9238795325112867385, 1.000000000000000000, 0.9238795325112867385, 1.000000000000000000, 0.9238795325112867385, 1.000000000000000000, 0.9238795325112867385, 1.000000000000000000, 0.9238795325112867385, 1.000000000000000000, 0.9238795325112867385, 1.000000000000000000, 0.9238795325112867385, 1.000000000000000000, 0.9238795325112867385, 1.000000000000000000, 0.9238795325112867385, 1.000000000000000000, 0.9238795325112867385, 1.000000000000000000, 0.9238795325112867385, 1.000000000000000000, 0.9238795325112867385, 1.000000000000000000, 0.9238795325112867385, 1.000000000000000000, 0.9238795325112867385, 1.000000000000000000, 0.9238795325112867385, 1.000000000000000000, 0.9238795325112867385, 1.000000000000000000, 0.9238795325112867385, 1.000000000000000000, 0.9238795325112867385, 1.000000000000000000, 0.9238795325112867385, 1.000000000000000000, 0.9238795325112867385, 1.000000000000000000, 0.9238795325112867385, 1.000000000000000000, 0.9238795325112867385, 1.000000000000000000, 0.9238795325112867385, 1.000000000000000000, 0.9238795325112867385, 1.000000000000000000, 0.9238795325112867385, 1.000000000000000000, 0.9238795325112867385, 1.000000000000000000, 0.9238795325112867385, 1.000000000000000000, 0.9238795325112867385, 1.000000000000000000, 0.9238795325112867385, 1.000000000000000000, 0.9238795325112867385, 1.000000000000000000, 0.9238795325112867385, 1.000000000000000000) ) ) 
 REPRESENTATION_ITEM ( '' )  SURFACE ( )  );
#20810=CARTESIAN_POINT ( 'NONE',  ( 13.31250000000012612, -0.8284271247460553989, 1.999999999999911626 ) ) ;
#20833=CARTESIAN_POINT ( 'NONE',  ( 19.00000000000020961, 2.000000000000223821, -5.551115123125782702E-14 ) ) ;
#20839=( LENGTH_UNIT ( ) NAMED_UNIT ( * ) SI_UNIT ( .MILLI., .METRE. ) );
#20851=ORIENTED_EDGE ( 'NONE', *, *, #10093, .F. ) ;
#20863=CARTESIAN_POINT ( 'NONE',  ( 13.64882486540520290, 2.500000000000205169, -1.035533905932809473 ) ) ;
#20866=CARTESIAN_POINT ( 'NONE',  ( 12.25000000000014921, -1.873492889144845464, -1.873492889145123019 ) ) ;
#20868=CARTESIAN_POINT ( 'NONE',  ( 12.71132486540518869, 2.500000000000002220, 0.000000000000000000 ) ) ;
#20880=CARTESIAN_POINT ( 'NONE',  ( 21.18750000000013500, 1.097466725451679892, -2.649519052838298805 ) ) ;
#20882=EDGE_CURVE ( 'NONE', #4865, #886, #4543, .T. ) ;
#20889=CARTESIAN_POINT ( 'NONE',  ( 10.87499999999996803, 1.414213562373312083, -1.414213562373145550 ) ) ;
#20893=CIRCLE ( 'NONE', #28697, 1.999999999999998224 ) ;
#20909=CARTESIAN_POINT ( 'NONE',  ( 22.93749999999999289, -1.097466725451499370, 2.649519052838358757 ) ) ;
#20914=CARTESIAN_POINT ( 'NONE',  ( 2.081668171172167281E-16, 3.582034040661430693E-16, -2.499999999999999112 ) ) ;
#20917=CARTESIAN_POINT ( 'NONE',  ( 16.96132486540522066, 1.110223024625156540E-13, 2.500000000000002220 ) ) ;
#20923=EDGE_CURVE ( 'NONE', #22647, #11887, #12426, .T. ) ;
#20925=CARTESIAN_POINT ( 'NONE',  ( 11.56250000000000000, 1.097466725451619718, 2.649519052838478661 ) ) ;
#20927=CARTESIAN_POINT ( 'NONE',  ( 14.78867513459480776, -2.500000000000002220, -5.551115123125782702E-14 ) ) ;
#20928=CARTESIAN_POINT ( 'NONE',  ( 23.12500000000003553, 1.414213562373090038, 1.414213562373034527 ) ) ;
#20955=CARTESIAN_POINT ( 'NONE',  ( 14.39882486540531303, -1.035533905932568999, -2.499999999999904521 ) ) ;
#20961=CARTESIAN_POINT ( 'NONE',  ( 13.68750000000000178, -0.8284271247459350507, -2.000000000000091926 ) ) ;
#20964=CARTESIAN_POINT ( 'NONE',  ( 10.00000000000015099, 0.5728653053451536747, -2.302908512320128942 ) ) ;
#20987=CARTESIAN_POINT ( 'NONE',  ( -2.081668171172168020E-16, -5.204170427930420051E-17, 2.499999999999999112 ) ) ;
#20989=CARTESIAN_POINT ( 'NONE',  ( 19.31250000000010303, -0.8284271247459350507, 2.000000000000091926 ) ) ;
#21022=CARTESIAN_POINT ( 'NONE',  ( 12.12500000000010836, -2.649519052838111843, -5.551115123125782702E-14 ) ) ;
#21040=CARTESIAN_POINT ( 'NONE',  ( 20.50000000000012790, 1.873492889145011997, 1.873492889144734441 ) ) ;
#21049=CARTESIAN_POINT ( 'NONE',  ( 23.46132486540525264, 1.110223024625156540E-13, -2.500000000000002220 ) ) ;
#21058=CARTESIAN_POINT ( 'NONE',  ( 22.31250000000015277, -1.097466725451439196, -2.649519052838358757 ) ) ;
#21061=CARTESIAN_POINT ( 'NONE',  ( 18.33632486540526330, -1.767766952966265404, -1.767766952966542959 ) ) ;
#21068=ORIENTED_EDGE ( 'NONE', *, *, #15426, .F. ) ;
#21069=CARTESIAN_POINT ( 'NONE',  ( 22.10117513459489302, 1.035533905932869425, -2.500000000000024425 ) ) ;
#21072=VERTEX_POINT ( 'NONE', #10722 ) ;
#21078=CARTESIAN_POINT ( 'NONE',  ( 11.12500000000010658, 1.665334536937734811E-13, -2.649519052838444910 ) ) ;
#21080=CARTESIAN_POINT ( 'NONE',  ( 18.50000000000012790, -1.999999999999835243, 0.000000000000000000 ) ) ;
#21084=CARTESIAN_POINT ( 'NONE',  ( 11.85117513459488592, -2.499999999999964473, -1.035533905932749299 ) ) ;
#21118=CARTESIAN_POINT ( 'NONE',  ( 11.96132486540524198, 1.110223024625156540E-13, 2.499999999999835687 ) ) ;
#21136=CARTESIAN_POINT ( 'NONE',  ( 18.06250000000005684, 2.000000000000151879, 0.8284271247461152399 ) ) ;
#21147=CARTESIAN_POINT ( 'NONE',  ( 19.37500000000019895, -1.414213562372979016, 1.414213562373034527 ) ) ;
#21162=DIRECTION ( 'NONE',  ( 0.000000000000000000, 8.673617379884043361E-16, 1.000000000000000000 ) ) ;
#21172=CARTESIAN_POINT ( 'NONE',  ( 10.25000000000012079, -1.873492889144845464, -1.873492889144956486 ) ) ;
#21179=CARTESIAN_POINT ( 'NONE',  ( 9.687499999999998224, -0.8284271247461152399, -1.999999999999971800 ) ) ;
#21188=CARTESIAN_POINT ( 'NONE',  ( 22.25000000000004619, 1.873492889145123019, -1.873492889144956486 ) ) ;
#21190=ORIENTED_EDGE ( 'NONE', *, *, #27158, .F. ) ;
#21211=CARTESIAN_POINT ( 'NONE',  ( 21.62500000000017053, 2.649519052838555933, -5.551115123125782702E-14 ) ) ;
#21216=LINE ( 'NONE', #12025, #7454 ) ;
#21219=CARTESIAN_POINT ( 'NONE',  ( 22.33632486540521001, -1.767766952966320915, -1.767766952966542959 ) ) ;
#21234=CARTESIAN_POINT ( 'NONE',  ( 12.03867513459491789, 1.665334536937734811E-13, -2.500000000000057732 ) ) ;
#21235=CARTESIAN_POINT ( 'NONE',  ( 12.97617513459487171, -1.035533905932629173, -2.500000000000084821 ) ) ;
#21236=( LENGTH_UNIT ( ) NAMED_UNIT ( * ) SI_UNIT ( .MILLI., .METRE. ) );
#21237=CARTESIAN_POINT ( 'NONE',  ( 24.79215710450393928, -1.034327703891616990, -1.956437050582624071 ) ) ;
#21282=CARTESIAN_POINT ( 'NONE',  ( 16.43750000000008527, -1.999999999999851674, 0.8284271247461753029 ) ) ;
#21292=CARTESIAN_POINT ( 'NONE',  ( 20.00000000000004619, 2.000000000000057288, -5.551115123125782702E-14 ) ) ;
#21296=CARTESIAN_POINT ( 'NONE',  ( 16.06250000000017764, -1.097466725451439196, -2.649519052838478661 ) ) ;
#21317=CARTESIAN_POINT ( 'NONE',  ( 24.81250000000011724, 0.8284271247463557142, -2.000000000000091926 ) ) ;
#21322=CARTESIAN_POINT ( 'NONE',  ( 20.28867513459483973, 2.500000000000002220, 0.000000000000000000 ) ) ;
#21333=CARTESIAN_POINT ( 'NONE',  ( 19.62500000000011369, 1.665334536937734811E-13, 2.649519052838278377 ) ) ;
#21357=CARTESIAN_POINT ( 'NONE',  ( 18.31250000000011724, -1.097466725451439196, -2.649519052838419153 ) ) ;
#21369=PRODUCT_DEFINITION ( 'UNKNOWN', '', #21764, #2654 ) ;
#21381=CARTESIAN_POINT ( 'NONE',  ( 17.68750000000009592, -0.8284271247460552878, -1.999999999999971800 ) ) ;
#21386=CARTESIAN_POINT ( 'NONE',  ( 22.53867513459501026, 1.110223024625156540E-13, 2.499999999999835687 ) ) ;
#21387=CARTESIAN_POINT ( 'NONE',  ( 12.46132486540529882, 1.110223024625156540E-13, -2.500000000000057732 ) ) ;
#21388=CARTESIAN_POINT ( 'NONE',  ( 23.03867513459492855, 2.220446049250313081E-13, -2.500000000000057732 ) ) ;
#21391=DIRECTION ( 'NONE',  ( -8.326672684688675286E-17, -2.081668171172168821E-17, 1.000000000000000000 ) ) ;
#21398=DIRECTION ( 'NONE',  ( 1.000000000000000000, 1.665334536937731113E-16, 8.326672684688674053E-17 ) ) ;
#21402=SURFACE_STYLE_FILL_AREA ( #26430 ) ;
#21445=CARTESIAN_POINT ( 'NONE',  ( 20.50000000000015632, -1.999999999999890754, -5.551115123125782702E-14 ) ) ;
#21490=CARTESIAN_POINT ( 'NONE',  ( 17.18750000000010303, 1.097466725451679892, -2.649519052838358757 ) ) ;
#21514=CARTESIAN_POINT ( 'NONE',  ( 17.00000000000007105, -1.873492889144845464, 1.873492889144845464 ) ) ;
#21532=CARTESIAN_POINT ( 'NONE',  ( 12.56249999999998579, 1.097466725451619718, 2.649519052838178457 ) ) ;
#21533=CARTESIAN_POINT ( 'NONE',  ( 18.96132486540530593, 1.110223024625156540E-13, 2.499999999999724665 ) ) ;
#21535=CARTESIAN_POINT ( 'NONE',  ( 18.93750000000016698, 2.000000000000091926, -0.8284271247462354770 ) ) ;
#21539=CARTESIAN_POINT ( 'NONE',  ( 23.03867513459492855, 2.220446049250313081E-13, -2.500000000000057732 ) ) ;
#21541=CARTESIAN_POINT ( 'NONE',  ( 15.28867513459483618, 2.500000000000113243, -1.665334536937734811E-13 ) ) ;
#21546=FACE_OUTER_BOUND ( 'NONE', #20075, .T. ) ;
#21550=CARTESIAN_POINT ( 'NONE',  ( 0.000000000000000000, 0.000000000000000000, 0.000000000000000000 ) ) ;
#21552=ORIENTED_EDGE ( 'NONE', *, *, #22293, .T. ) ;
#21554=CARTESIAN_POINT ( 'NONE',  ( 12.46132486540529882, 1.110223024625156540E-13, -2.500000000000057732 ) ) ;
#21555=CARTESIAN_POINT ( 'NONE',  ( 11.81250000000006040, 0.8284271247463557142, -2.000000000000031530 ) ) ;
#21560=VERTEX_POINT ( 'NONE', #23103 ) ;
#21594=CARTESIAN_POINT ( 'NONE',  ( 20.18750000000014566, 0.8284271247463557142, 1.999999999999911626 ) ) ;
#21599=CARTESIAN_POINT ( 'NONE',  ( 15.87500000000016698, -2.649519052838000821, -1.110223024625156540E-13 ) ) ;
#21601=ORIENTED_EDGE ( 'NONE', *, *, #19113, .T. ) ;
#21617=CARTESIAN_POINT ( 'NONE',  ( 24.16367513459488592, 1.767766952966487448, -1.767766952966431937 ) ) ;
#21622=CARTESIAN_POINT ( 'NONE',  ( 23.75000000000013145, 1.665334536937734811E-13, -2.000000000000057288 ) ) ;
#21638=CARTESIAN_POINT ( 'NONE',  ( 2.081668171172167281E-16, 3.582034040661430693E-16, -2.499999999999999112 ) ) ;
#21644=ADVANCED_FACE ( 'NONE', ( #8812 ), #24918, .F. ) ;
#21661=CARTESIAN_POINT ( 'NONE',  ( 18.93750000000004619, -1.097466725451439196, 2.649519052838178457 ) ) ;
#21667=CARTESIAN_POINT ( 'NONE',  ( 17.16367513459499250, 1.767766952966431937, -1.767766952966431937 ) ) ;
#21668=CARTESIAN_POINT ( 'NONE',  ( 22.64882486540529172, 2.500000000000144773, -1.035533905932809473 ) ) ;
#21670=CARTESIAN_POINT ( 'NONE',  ( 22.28867513459495342, 2.500000000000113243, -1.665334536937734811E-13 ) ) ;
#21678=CARTESIAN_POINT ( 'NONE',  ( 24.21132486540530948, -2.499999999999946709, -2.220446049250313081E-13 ) ) ;
#21706=CARTESIAN_POINT ( 'NONE',  ( 20.52382486540534856, 1.035533905932809473, -2.499999999999904521 ) ) ;
#21709=ADVANCED_FACE ( 'NONE', ( #7256 ), #23702, .T. ) ;
#21736=CARTESIAN_POINT ( 'NONE',  ( 17.75000000000015632, 1.110223024625156540E-13, -2.000000000000001776 ) ) ;
#21747=CARTESIAN_POINT ( 'NONE',  ( 19.50000000000009948, -1.999999999999835243, 0.000000000000000000 ) ) ;
#21752=CARTESIAN_POINT ( 'NONE',  ( 0.000000000000000000, 0.000000000000000000, 0.000000000000000000 ) ) ;
#21764=PRODUCT_DEFINITION_FORMATION_WITH_SPECIFIED_SOURCE ( 'ANY', '', #10914, .NOT_KNOWN. ) ;
#21770=DIRECTION ( 'NONE',  ( -1.000000000000000000, -1.665334536937731113E-16, 1.526556658859586792E-16 ) ) ;
#21775=ORIENTED_EDGE ( 'NONE', *, *, #27158, .T. ) ;
#21782=CARTESIAN_POINT ( 'NONE',  ( 20.25000000000009948, 1.873492889145067508, -1.873492889144956486 ) ) ;
#21798=CARTESIAN_POINT ( 'NONE',  ( 23.25000000000004974, 5.551115123125782702E-14, 1.999999999999946265 ) ) ;
#21813=CARTESIAN_POINT ( 'NONE',  ( 24.82006884940611613, 1.953411417485240831, -0.9991708543551893751 ) ) ;
#21816=EDGE_LOOP ( 'NONE', ( #11194, #11142, #15931, #4681 ) ) ;
#21819=CARTESIAN_POINT ( 'NONE',  ( 11.00000000000014921, 2.000000000000112799, 0.000000000000000000 ) ) ;
#21827=CARTESIAN_POINT ( 'NONE',  ( 14.56249999999998934, -1.999999999999851674, -0.8284271247462354770 ) ) ;
#21832=CARTESIAN_POINT ( 'NONE',  ( 15.35117513459492677, 2.500000000000144773, 1.035533905932689347 ) ) ;
#21869=( BOUNDED_CURVE ( )  B_SPLINE_CURVE ( 2, ( #11426, #27643, #18031, #27487, #29508, #4315, #20158, #22917, #11263 ),
 .UNSPECIFIED., .F., .T. ) 
 B_SPLINE_CURVE_WITH_KNOTS ( ( 3, 2, 2, 2, 3 ),
 ( 0.1718750000000000000, 0.1796875000000000000, 0.1875000000000000000, 0.1953125000000000000, 0.2031250000000000000 ),
 .UNSPECIFIED. ) 
 CURVE ( )  GEOMETRIC_REPRESENTATION_ITEM ( )  RATIONAL_B_SPLINE_CURVE ( ( 1.000000000000000000, 0.9238795325112867385, 1.000000000000000000, 0.9238795325112867385, 1.000000000000000000, 0.9238795325112867385, 1.000000000000000000, 0.9238795325112867385, 1.000000000000000000 ) ) 
 REPRESENTATION_ITEM ( '' )  );
#21878=ORIENTED_EDGE ( 'NONE', *, *, #5752, .T. ) ;
#21882=CIRCLE ( 'NONE', #10138, 1.999999999999998224 ) ;
#21886=EDGE_LOOP ( 'NONE', ( #11678, #28971, #15735 ) ) ;
#21891=CARTESIAN_POINT ( 'NONE',  ( 17.25000000000001421, 1.665334536937734811E-13, 2.000000000000001776 ) ) ;
#21894=ORIENTED_EDGE ( 'NONE', *, *, #9688, .T. ) ;
#21896=CARTESIAN_POINT ( 'NONE',  ( 15.56250000000015810, 1.097466725451679892, 2.649519052838298805 ) ) ;
#21927=ORIENTED_EDGE ( 'NONE', *, *, #9674, .F. ) ;
#21945=LINE ( 'NONE', #8089, #12359 ) ;
#21946=EDGE_CURVE ( 'NONE', #11887, #28765, #25153, .T. ) ;
#21953=ORIENTED_EDGE ( 'NONE', *, *, #9361, .F. ) ;
#21961=VERTEX_POINT ( 'NONE', #1966 ) ;
#21973=CARTESIAN_POINT ( 'NONE',  ( 16.25000000000009948, 1.665334536937734811E-13, 2.000000000000001776 ) ) ;
#21987=CARTESIAN_POINT ( 'NONE',  ( 13.46132486540532724, 1.665334536937734811E-13, -2.500000000000057732 ) ) ;
#22024=CARTESIAN_POINT ( 'NONE',  ( 15.31250000000006928, -0.8284271247461753029, 1.999999999999911626 ) ) ;
#22035=CARTESIAN_POINT ( 'NONE',  ( 17.87500000000008527, 1.414213562373312083, -1.414213562373145550 ) ) ;
#22038=EDGE_CURVE ( 'NONE', #12351, #2749, #10477, .T. ) ;
#22048=( NAMED_UNIT ( * ) SI_UNIT ( $, .STERADIAN. ) SOLID_ANGLE_UNIT ( ) );
#22075=ADVANCED_FACE ( 'NONE', ( #12425 ), #19306, .T. ) ;
#22088=DIRECTION ( 'NONE',  ( -8.326672684688675286E-17, -2.081668171172168821E-17, 1.000000000000000000 ) ) ;
#22093=FACE_OUTER_BOUND ( 'NONE', #11768, .T. ) ;
#22096=CARTESIAN_POINT ( 'NONE',  ( 24.68750000000014566, -0.8284271247460553989, -2.000000000000151879 ) ) ;
#22105=CARTESIAN_POINT ( 'NONE',  ( 14.75000000000012434, 1.873492889145067508, 1.873492889144734441 ) ) ;
#22115=ORIENTED_EDGE ( 'NONE', *, *, #7278, .T. ) ;
#22125=CARTESIAN_POINT ( 'NONE',  ( 15.37500000000011013, -1.414213562373034527, 1.414213562373034527 ) ) ;
#22136=( BOUNDED_CURVE ( )  B_SPLINE_CURVE ( 2, ( #1721, #6320, #18188, #25059, #16060, #2035, #3857, #18345, #11277 ),
 .UNSPECIFIED., .F., .T. ) 
 B_SPLINE_CURVE_WITH_KNOTS ( ( 3, 2, 2, 2, 3 ),
 ( 0.1406250000000000000, 0.1484375000000000000, 0.1562500000000000000, 0.1640625000000000000, 0.1718750000000000000 ),
 .UNSPECIFIED. ) 
 CURVE ( )  GEOMETRIC_REPRESENTATION_ITEM ( )  RATIONAL_B_SPLINE_CURVE ( ( 1.000000000000000000, 0.9238795325112867385, 1.000000000000000000, 0.9238795325112867385, 1.000000000000000000, 0.9238795325112867385, 1.000000000000000000, 0.9238795325112867385, 1.000000000000000000 ) ) 
 REPRESENTATION_ITEM ( '' )  );
#22145=CARTESIAN_POINT ( 'NONE',  ( 11.03867513459494454, 1.665334536937734811E-13, -2.500000000000113243 ) ) ;
#22146=CARTESIAN_POINT ( 'NONE',  ( 10.50000000000003730, -1.999999999999835243, 0.000000000000000000 ) ) ;
#22156=CARTESIAN_POINT ( 'NONE',  ( 25.31250000000007816, 2.649519052838419153, -1.097466725451439196 ) ) ;
#22160=DIRECTION ( 'NONE',  ( -1.000000000000000000, -1.665334536937731113E-16, 1.526556658859586792E-16 ) ) ;
#22179=CARTESIAN_POINT ( 'NONE',  ( 15.87500000000008349, 1.414213562373201061, -1.414213562373090038 ) ) ;
#22187=EDGE_LOOP ( 'NONE', ( #13808, #14337, #13732, #19477 ) ) ;
#22191=CARTESIAN_POINT ( 'NONE',  ( 16.62500000000013856, -1.414213562372867994, -1.414213562373145550 ) ) ;
#22195=CARTESIAN_POINT ( 'NONE',  ( 13.62500000000005329, 5.551115123125782702E-14, 2.649519052838167354 ) ) ;
#22198=FACE_OUTER_BOUND ( 'NONE', #443, .T. ) ;
#22217=( BOUNDED_CURVE ( )  B_SPLINE_CURVE ( 2, ( #25381, #20955, #18361, #25542, #13608, #13454, #27834, #22800, #2209 ),
 .UNSPECIFIED., .F., .T. ) 
 B_SPLINE_CURVE_WITH_KNOTS ( ( 3, 2, 2, 2, 3 ),
 ( 0.6406250000000000000, 0.6484375000000000000, 0.6562500000000000000, 0.6640625000000000000, 0.6718750000000000000 ),
 .UNSPECIFIED. ) 
 CURVE ( )  GEOMETRIC_REPRESENTATION_ITEM ( )  RATIONAL_B_SPLINE_CURVE ( ( 1.000000000000000000, 0.9238795325112867385, 1.000000000000000000, 0.9238795325112867385, 1.000000000000000000, 0.9238795325112867385, 1.000000000000000000, 0.9238795325112867385, 1.000000000000000000 ) ) 
 REPRESENTATION_ITEM ( '' )  );
#22239=CYLINDRICAL_SURFACE ( 'NONE', #3199, 2.499999999999999112 ) ;
#22253=CARTESIAN_POINT ( 'NONE',  ( 13.75000000000012257, 1.873492889145067508, 1.873492889144734441 ) ) ;
#22265=ORIENTED_EDGE ( 'NONE', *, *, #7099, .F. ) ;
#22274=CARTESIAN_POINT ( 'NONE',  ( 19.96132486540530593, 5.551115123125782702E-14, 2.500000000000002220 ) ) ;
#22276=CARTESIAN_POINT ( 'NONE',  ( 16.50000000000004263, -1.999999999999835243, 0.000000000000000000 ) ) ;
#22292=CARTESIAN_POINT ( 'NONE',  ( 24.18750000000012079, -2.649519052838238409, -1.097466725451499370 ) ) ;
#22293=EDGE_CURVE ( 'NONE', #15054, #18896, #27126, .T. ) ;
#22295=CARTESIAN_POINT ( 'NONE',  ( 16.77382486540527751, 2.500000000000144773, 1.035533905932749299 ) ) ;
#22307=CARTESIAN_POINT ( 'NONE',  ( 24.68750000000011724, -1.097466725451379244, 2.649519052838238409 ) ) ;
#22323=CARTESIAN_POINT ( 'NONE',  ( 16.28867513459492145, 2.500000000000002220, 0.000000000000000000 ) ) ;
#22333=CARTESIAN_POINT ( 'NONE',  ( 16.12500000000002842, 1.414213562373201061, 1.414213562373034527 ) ) ;
#22343=CARTESIAN_POINT ( 'NONE',  ( 15.93749999999996980, 2.000000000000091926, -0.8284271247462955401 ) ) ;
#22347=CARTESIAN_POINT ( 'NONE',  ( 15.31250000000006928, 2.649519052838478661, -1.097466725451679892 ) ) ;
#22375=VECTOR ( 'NONE', #18907, 1000.000000000000000 ) ;
#22376=CARTESIAN_POINT ( 'NONE',  ( 24.91299458739716854, 1.355376207975084402, -1.592815096892554516 ) ) ;
#22378=VERTEX_POINT ( 'NONE', #5907 ) ;
#22386=CARTESIAN_POINT ( 'NONE',  ( 21.53867513459484329, 0.000000000000000000, 2.500000000000002220 ) ) ;
#22400=EDGE_CURVE ( 'NONE', #3562, #23786, #20678, .T. ) ;
#22407=CARTESIAN_POINT ( 'NONE',  ( 16.43750000000011013, 1.097466725451619718, -2.649519052838298805 ) ) ;
#22411=( BOUNDED_CURVE ( )  B_SPLINE_CURVE ( 2, ( #25908, #16587, #256, #9639, #7467, #20863, #2418, #16879, #26199 ),
 .UNSPECIFIED., .F., .T. ) 
 B_SPLINE_CURVE_WITH_KNOTS ( ( 3, 2, 2, 2, 3 ),
 ( 0.6718750000000000000, 0.6796875000000000000, 0.6875000000000000000, 0.6953125000000000000, 0.7031250000000000000 ),
 .UNSPECIFIED. ) 
 CURVE ( )  GEOMETRIC_REPRESENTATION_ITEM ( )  RATIONAL_B_SPLINE_CURVE ( ( 1.000000000000000000, 0.9238795325112867385, 1.000000000000000000, 0.9238795325112867385, 1.000000000000000000, 0.9238795325112867385, 1.000000000000000000, 0.9238795325112867385, 1.000000000000000000 ) ) 
 REPRESENTATION_ITEM ( '' )  );
#22418=CARTESIAN_POINT ( 'NONE',  ( 24.63750948478215363, 1.344396243822401082, -1.946671111007823862 ) ) ;
#22433=CARTESIAN_POINT ( 'NONE',  ( 16.81250000000007816, 0.8284271247462955401, -2.000000000000091926 ) ) ;
#22445=EDGE_CURVE ( 'NONE', #15054, #566, #30030, .T. ) ;
#22450=CARTESIAN_POINT ( 'NONE',  ( 23.37500000000011724, 1.665334536937734811E-13, -2.649519052838333888 ) ) ;
#22476=CARTESIAN_POINT ( 'NONE',  ( 24.53037769546397584, -0.1516104150550960927, 2.469622304536084112 ) ) ;
#22494=CARTESIAN_POINT ( 'NONE',  ( 16.18750000000014566, 0.8284271247462955401, 2.000000000000031530 ) ) ;
#22504=CARTESIAN_POINT ( 'NONE',  ( 18.93750000000016698, 2.000000000000091926, -0.8284271247462354770 ) ) ;
#22523=CARTESIAN_POINT ( 'NONE',  ( 24.41367513459491434, 1.767766952966431937, 1.767766952966320915 ) ) ;
#22542=CARTESIAN_POINT ( 'NONE',  ( 17.96132486540527751, 1.110223024625156540E-13, 2.499999999999946709 ) ) ;
#22561=CARTESIAN_POINT ( 'NONE',  ( 24.50000000000010658, 5.551115123125782702E-14, -5.551115123125782702E-14 ) ) ;
#22564=CARTESIAN_POINT ( 'NONE',  ( 15.93750000000009059, -1.097466725451439196, 2.649519052838178457 ) ) ;
#22570=EDGE_CURVE ( 'NONE', #27492, #11541, #23592, .T. ) ;
#22603=CARTESIAN_POINT ( 'NONE',  ( 23.31250000000007461, -1.097466725451379244, -2.649519052838478661 ) ) ;
#22610=CARTESIAN_POINT ( 'NONE',  ( 10.60117513459496408, -1.035533905932629173, 2.499999999999964473 ) ) ;
#22615=CARTESIAN_POINT ( 'NONE',  ( 10.00000000000009237, 2.022486306914408782, 0.1720805556212724186 ) ) ;
#22625=CARTESIAN_POINT ( 'NONE',  ( 24.12500000000009237, 1.414213562373201061, 1.414213562373034527 ) ) ;
#22633=CARTESIAN_POINT ( 'NONE',  ( 14.16367513459490546, 1.767766952966487448, -1.767766952966487448 ) ) ;
#22639=PRESENTATION_STYLE_ASSIGNMENT (( #13297 ) ) ;
#22647=VERTEX_POINT ( 'NONE', #8800 ) ;
#22653=CARTESIAN_POINT ( 'NONE',  ( 14.12500000000013678, 1.414213562373201061, 1.414213562373034527 ) ) ;
#22657=CARTESIAN_POINT ( 'NONE',  ( 14.31250000000002132, 2.649519052838298805, -1.097466725451559322 ) ) ;
#22674=CARTESIAN_POINT ( 'NONE',  ( 20.93750000000008171, 2.000000000000212275, -0.8284271247463557142 ) ) ;
#22712=CARTESIAN_POINT ( 'NONE',  ( 15.43750000000003730, 1.097466725451559322, -2.649519052838298805 ) ) ;
#22735=CARTESIAN_POINT ( 'NONE',  ( 20.27382486540532014, -2.499999999999844569, -1.035533905932809473 ) ) ;
#22737=CARTESIAN_POINT ( 'NONE',  ( 12.06249999999996447, 2.000000000000091926, 0.8284271247461753029 ) ) ;
#22751=AXIS2_PLACEMENT_3D ( 'NONE', #21550, #4933, #25529 ) ;
#22755=CARTESIAN_POINT ( 'NONE',  ( 17.60117513459492500, -1.035533905932629173, 2.499999999999784173 ) ) ;
#22760=CARTESIAN_POINT ( 'NONE',  ( 9.812500000000115463, 0.8284271247462955401, -2.000000000000091926 ) ) ;
#22770=CARTESIAN_POINT ( 'NONE',  ( 24.62500000000012079, -1.414213562372923505, -1.414213562373145550 ) ) ;
#22780=ADVANCED_FACE ( 'NONE', ( #2187 ), #1612, .T. ) ;
#22785=CARTESIAN_POINT ( 'NONE',  ( 14.10117513459491612, 1.035533905932929599, -2.500000000000024425 ) ) ;
#22792=ORIENTED_EDGE ( 'NONE', *, *, #3431, .F. ) ;
#22797=CARTESIAN_POINT ( 'NONE',  ( 13.37500000000019185, -1.414213562372979016, 1.414213562372979016 ) ) ;
#22800=CARTESIAN_POINT ( 'NONE',  ( 14.02382486540528816, -1.035533905932568999, 2.499999999999784173 ) ) ;
#22803=CARTESIAN_POINT ( 'NONE',  ( 12.06249999999996447, 2.000000000000091926, 0.8284271247461753029 ) ) ;
#22806=CARTESIAN_POINT ( 'NONE',  ( 10.00000000000014921, 0.7338214498545042597, -2.235074556132228274 ) ) ;
#22814=CARTESIAN_POINT ( 'NONE',  ( 19.16367513459482552, 1.767766952966376426, -1.767766952966431937 ) ) ;
#22818=EDGE_CURVE ( 'NONE', #7192, #11887, #2278, .T. ) ;
#22842=VERTEX_POINT ( 'NONE', #21388 ) ;
#22855=CARTESIAN_POINT ( 'NONE',  ( 23.58632486540529527, 1.767766952966431937, -1.767766952966431937 ) ) ;
#22864=CARTESIAN_POINT ( 'NONE',  ( 10.93750000000001066, -1.097466725451439196, 2.649519052838178457 ) ) ;
#22877=CARTESIAN_POINT ( 'NONE',  ( 24.31250000000012079, 2.649519052838419153, -1.097466725451559322 ) ) ;
#22886=ORIENTED_EDGE ( 'NONE', *, *, #27680, .T. ) ;
#22887=CARTESIAN_POINT ( 'NONE',  ( 11.68750000000000000, -0.8284271247461753029, -1.999999999999971800 ) ) ;
#22902=CARTESIAN_POINT ( 'NONE',  ( 22.37500000000014566, 1.665334536937734811E-13, -2.649519052838333888 ) ) ;
#22907=AXIS2_PLACEMENT_3D ( 'NONE', #17267, #26588, #937 ) ;
#22914=CARTESIAN_POINT ( 'NONE',  ( 10.00000000000014921, -0.4401475947494610241, 2.447530906695864150 ) ) ;
#22917=CARTESIAN_POINT ( 'NONE',  ( 21.52382486540530238, 1.035533905932929599, -2.499999999999964473 ) ) ;
#22923=CARTESIAN_POINT ( 'NONE',  ( 24.18750000000015277, 0.8284271247463557142, 2.000000000000031530 ) ) ;
#22950=CARTESIAN_POINT ( 'NONE',  ( 12.56250000000007638, -1.999999999999851674, -0.8284271247462354770 ) ) ;
#22959=CARTESIAN_POINT ( 'NONE',  ( 14.75000000000009592, 2.220446049250313081E-13, -2.000000000000057288 ) ) ;
#22962=CARTESIAN_POINT ( 'NONE',  ( 18.83632486540531659, 1.767766952966431937, 1.767766952966320915 ) ) ;
#22966=DIRECTION ( 'NONE',  ( -1.000000000000000000, -1.665334536937731113E-16, 1.526556658859586792E-16 ) ) ;
#22973=CARTESIAN_POINT ( 'NONE',  ( -2.081668171172168020E-16, -5.204170427930420051E-17, 2.499999999999999112 ) ) ;
#22983=CARTESIAN_POINT ( 'NONE',  ( 21.25000000000015632, 0.000000000000000000, 2.000000000000057288 ) ) ;
#22991=EDGE_CURVE ( 'NONE', #21072, #23786, #13457, .T. ) ;
#23017=CARTESIAN_POINT ( 'NONE',  ( 10.62500000000016165, 2.649519052838555933, 1.110223024625156540E-13 ) ) ;
#23019=CARTESIAN_POINT ( 'NONE',  ( 12.52382486540527751, 1.035533905932809473, -2.499999999999904521 ) ) ;
#23034=CARTESIAN_POINT ( 'NONE',  ( 22.93750000000013856, -2.649519052838178457, -1.097466725451559322 ) ) ;
#23044=ORIENTED_EDGE ( 'NONE', *, *, #6430, .T. ) ;
#23056=CARTESIAN_POINT ( 'NONE',  ( 10.41367513459478999, 1.767766952966376426, 1.767766952966376426 ) ) ;
#23061=CARTESIAN_POINT ( 'NONE',  ( 19.75000000000012790, 1.873492889145123019, 1.873492889144845464 ) ) ;
#23073=CARTESIAN_POINT ( 'NONE',  ( 17.14882486540524553, -2.499999999999904521, 1.035533905932749299 ) ) ;
#23084=CARTESIAN_POINT ( 'NONE',  ( 23.25000000000004974, 5.551115123125782702E-14, 1.999999999999946265 ) ) ;
#23103=CARTESIAN_POINT ( 'NONE',  ( 17.53867513459494987, 1.665334536937734811E-13, 2.499999999999946709 ) ) ;
#23115=ORIENTED_EDGE ( 'NONE', *, *, #5088, .T. ) ;
#23116=CARTESIAN_POINT ( 'NONE',  ( 14.00000000000006750, 2.000000000000112799, 0.000000000000000000 ) ) ;
#23128=CARTESIAN_POINT ( 'NONE',  ( 19.28867513459494987, 2.500000000000057732, -5.551115123125782702E-14 ) ) ;
#23143=CARTESIAN_POINT ( 'NONE',  ( 20.68750000000011369, -0.8284271247459952248, -1.999999999999971800 ) ) ;
#23144=CARTESIAN_POINT ( 'NONE',  ( 2.081668171172167281E-16, 3.582034040661430693E-16, -2.499999999999999112 ) ) ;
#23157=ORIENTED_EDGE ( 'NONE', *, *, #10974, .F. ) ;
#23161=LINE ( 'NONE', #16122, #8114 ) ;
#23170=EDGE_CURVE ( 'NONE', #29809, #1806, #23360, .T. ) ;
#23178=CARTESIAN_POINT ( 'NONE',  ( 11.31250000000009592, -1.097466725451379244, -2.649519052838478661 ) ) ;
#23180=CARTESIAN_POINT ( 'NONE',  ( 15.66367513459493388, -1.767766952966154381, 1.767766952966376426 ) ) ;
#23182=EDGE_CURVE ( 'NONE', #6843, #5319, #29533, .T. ) ;
#23193=CARTESIAN_POINT ( 'NONE',  ( 21.56250000000010303, 1.097466725451739622, 2.649519052838358757 ) ) ;
#23201=CARTESIAN_POINT ( 'NONE',  ( 11.00000000000014921, 2.000000000000112799, 0.000000000000000000 ) ) ;
#23217=VERTEX_POINT ( 'NONE', #11081 ) ;
#23218=CARTESIAN_POINT ( 'NONE',  ( 22.87500000000019895, 5.551115123125782702E-14, 2.649519052838333888 ) ) ;
#23230=CARTESIAN_POINT ( 'NONE',  ( 10.00000000000014744, 1.983323942878633561, 0.6855453763663131861 ) ) ;
#23239=CARTESIAN_POINT ( 'NONE',  ( 23.37500000000000711, -1.414213562373090038, 1.414213562373034527 ) ) ;
#23248=CARTESIAN_POINT ( 'NONE',  ( 24.83473542850078530, -0.1527816007967785494, -2.165264571499343482 ) ) ;
#23271=CARTESIAN_POINT ( 'NONE',  ( 12.00000000000012079, 2.000000000000112799, -1.665334536937734811E-13 ) ) ;
#23275=CARTESIAN_POINT ( 'NONE',  ( 10.00000000000015277, 1.172446178180804210, -1.967641972052887933 ) ) ;
#23298=CARTESIAN_POINT ( 'NONE',  ( 19.81250000000009237, 0.8284271247463557142, -2.000000000000091926 ) ) ;
#23325=CARTESIAN_POINT ( 'NONE',  ( 20.96132486540536277, 5.551115123125782702E-14, 2.500000000000002220 ) ) ;
#23332=CARTESIAN_POINT ( 'NONE',  ( 12.31250000000004974, -1.097466725451499370, -2.649519052838358757 ) ) ;
#23351=CARTESIAN_POINT ( 'NONE',  ( 20.75000000000012790, -1.873492889144789952, 1.873492889144845464 ) ) ;
#23360=LINE ( 'NONE', #9058, #23434 ) ;
#23370=CARTESIAN_POINT ( 'NONE',  ( 21.74999999999999289, 1.873492889144956486, 1.873492889144734441 ) ) ;
#23371=CARTESIAN_POINT ( 'NONE',  ( 18.03867513459492145, 1.665334536937734811E-13, -2.500000000000057732 ) ) ;
#23381=ORIENTED_EDGE ( 'NONE', *, *, #22991, .F. ) ;
#23382=CARTESIAN_POINT ( 'NONE',  ( 20.97617513459490723, -1.035533905932689347, -2.500000000000024425 ) ) ;
#23386=CARTESIAN_POINT ( 'NONE',  ( 11.06250000000009948, -1.097466725451439196, -2.649519052838478661 ) ) ;
#23388=CARTESIAN_POINT ( 'NONE',  ( 19.00000000000020961, 2.000000000000223821, -5.551115123125782702E-14 ) ) ;
#23394=CARTESIAN_POINT ( 'NONE',  ( 11.72617513459494809, -2.499999999999964473, 1.035533905932749299 ) ) ;
#23397=B_SPLINE_CURVE_WITH_KNOTS ( 'NONE', 3,
 ( #12475, #17522, #13086, #21813, #3194, #12620, #5799, #5497, #22418, #29304, #17223, #8259 ),
 .UNSPECIFIED., .F., .F.,
 ( 4, 2, 2, 2, 2, 4 ),
 ( 1.086937293533992048E-16, 0.0007621846814068694662, 0.001524369362813630079, 0.001905461703517011361, 0.002286554044220393076, 0.003048738725627156941 ),
 .UNSPECIFIED. ) ;
#23433=CARTESIAN_POINT ( 'NONE',  ( 0.000000000000000000, 0.000000000000000000, 0.000000000000000000 ) ) ;
#23434=VECTOR ( 'NONE', #4129, 1000.000000000000000 ) ;
#23439=AXIS2_PLACEMENT_3D ( 'NONE', #26026, #13959, #23742 ) ;
#23446=CARTESIAN_POINT ( 'NONE',  ( 18.25000000000009948, 1.110223024625156540E-13, 1.999999999999946265 ) ) ;
#23461=CARTESIAN_POINT ( 'NONE',  ( 22.50000000000010303, -1.999999999999835243, 0.000000000000000000 ) ) ;
#23473=DIRECTION ( 'NONE',  ( 1.000000000000000000, 1.665334536937731113E-16, -1.526556658859586792E-16 ) ) ;
#23481=CARTESIAN_POINT ( 'NONE',  ( 24.46132486540536632, 1.665334536937734811E-13, -2.500000000000002220 ) ) ;
#23484=CARTESIAN_POINT ( 'NONE',  ( 11.25000000000009237, -1.873492889144900975, -1.873492889145011997 ) ) ;
#23486=CARTESIAN_POINT ( 'NONE',  ( 9.999999999999841904, 2.000000000000057288, -4.274358644806852681E-12 ) ) ;
#23496=CARTESIAN_POINT ( 'NONE',  ( 24.25000000000021672, 1.873492889145067508, -1.873492889144956486 ) ) ;
#23517=ORIENTED_EDGE ( 'NONE', *, *, #18079, .F. ) ;
#23518=CARTESIAN_POINT ( 'NONE',  ( 22.62500000000008882, 2.649519052838444910, 0.000000000000000000 ) ) ;
#23523=ORIENTED_EDGE ( 'NONE', *, *, #9012, .T. ) ;
#23535=CARTESIAN_POINT ( 'NONE',  ( 12.00000000000012079, -1.873492889144789952, -1.873492889145011997 ) ) ;
#23537=CARTESIAN_POINT ( 'NONE',  ( 20.81250000000014211, 0.8284271247461753029, -2.000000000000091926 ) ) ;
#23544=CARTESIAN_POINT ( 'NONE',  ( 24.77133704109404277, -1.424057122634293959, -1.721093397680183656 ) ) ;
#23548=VECTOR ( 'NONE', #5218, 1000.000000000000114 ) ;
#23552=EDGE_CURVE ( 'NONE', #18896, #27181, #17610, .T. ) ;
#23591=CARTESIAN_POINT ( 'NONE',  ( 17.56250000000009592, -1.999999999999851674, -0.8284271247461753029 ) ) ;
#23592=LINE ( 'NONE', #11440, #2109 ) ;
#23603=CARTESIAN_POINT ( 'NONE',  ( 21.87500000000011724, 1.414213562373201061, -1.414213562373090038 ) ) ;
#23608=CARTESIAN_POINT ( 'NONE',  ( 16.12500000000005684, 1.665334536937734811E-13, -2.649519052838444910 ) ) ;
#23610=ORIENTED_EDGE ( 'NONE', *, *, #17078, .T. ) ;
#23612=AXIS2_PLACEMENT_3D ( 'NONE', #28210, #18888, #408 ) ;
#23636=DIRECTION ( 'NONE',  ( -1.000000000000000000, -1.665334536937731113E-16, 1.526556658859586792E-16 ) ) ;
#23645=CARTESIAN_POINT ( 'NONE',  ( 24.18750000000006395, 1.097466725451559322, -2.649519052838358757 ) ) ;
#23652=CIRCLE ( 'NONE', #5451, 2.499999999999998224 ) ;
#23682=CARTESIAN_POINT ( 'NONE',  ( 11.68750000000011902, -1.097466725451379244, 2.649519052838238409 ) ) ;
#23685=CARTESIAN_POINT ( 'NONE',  ( 18.00000000000012790, 2.000000000000112799, 0.000000000000000000 ) ) ;
#23698=CARTESIAN_POINT ( 'NONE',  ( 15.83632486540537165, 1.767766952966542959, 1.767766952966209892 ) ) ;
#23699=CARTESIAN_POINT ( 'NONE',  ( 14.53867513459486460, 1.665334536937734811E-13, 2.499999999999835687 ) ) ;
#23702=CYLINDRICAL_SURFACE ( 'NONE', #22751, 2.499999999999999112 ) ;
#23717=DIRECTION ( 'NONE',  ( -1.000000000000000000, -1.665334536937731113E-16, 1.526556658859586792E-16 ) ) ;
#23740=CARTESIAN_POINT ( 'NONE',  ( 17.12500000000005684, 1.414213562373090038, 1.414213562373201061 ) ) ;
#23742=DIRECTION ( 'NONE',  ( -8.326672684688675286E-17, -2.081668171172168821E-17, 1.000000000000000000 ) ) ;
#23749=CARTESIAN_POINT ( 'NONE',  ( 19.18750000000004263, 0.8284271247462955401, 2.000000000000031530 ) ) ;
#23769=CARTESIAN_POINT ( 'NONE',  ( 24.68750000000014566, -0.8284271247460552878, -2.000000000000151879 ) ) ;
#23773=CARTESIAN_POINT ( 'NONE',  ( 10.00000000000014388, 2.023420126299062982, -0.3429612746322239780 ) ) ;
#23783=CARTESIAN_POINT ( 'NONE',  ( 17.31250000000004263, 2.649519052838419153, -1.097466725451439196 ) ) ;
#23786=VERTEX_POINT ( 'NONE', #15936 ) ;
#23806=VERTEX_POINT ( 'NONE', #21118 ) ;
#23807=CARTESIAN_POINT ( 'NONE',  ( 18.87500000000014211, 1.110223024625156540E-13, 2.649519052838056332 ) ) ;
#23814=CARTESIAN_POINT ( 'NONE',  ( 22.96132486540528106, 1.665334536937734811E-13, 2.499999999999946709 ) ) ;
#23828=CARTESIAN_POINT ( 'NONE',  ( 19.39882486540527040, -1.035533905932568999, -2.499999999999904521 ) ) ;
#23829=EDGE_LOOP ( 'NONE', ( #8653, #10828, #9570, #26109 ) ) ;
#23830=CARTESIAN_POINT ( 'NONE',  ( 20.06250000000006395, 2.000000000000151879, 0.8284271247461753029 ) ) ;
#23836=CARTESIAN_POINT ( 'NONE',  ( 11.96132486540524198, 1.110223024625156540E-13, 2.499999999999835687 ) ) ;
#23848=CARTESIAN_POINT ( 'NONE',  ( 24.99999999999999289, 1.110223024625156540E-13, -2.220446049250313081E-13 ) ) ;
#23878=CYLINDRICAL_SURFACE ( 'NONE', #1583, 2.499999999999999112 ) ;
#23879=CARTESIAN_POINT ( 'NONE',  ( 17.62500000000008527, -1.414213562372923505, -1.414213562373145550 ) ) ;
#23891=CARTESIAN_POINT ( 'NONE',  ( 23.12500000000003553, 1.414213562373090038, 1.414213562373034527 ) ) ;
#23916=CARTESIAN_POINT ( 'NONE',  ( 24.06250000000009592, 2.000000000000091926, 0.8284271247461152399 ) ) ;
#23928=( BOUNDED_CURVE ( )  B_SPLINE_CURVE ( 2, ( #25918, #16596, #4866, #14296, #27189, #25774, #13269, #1702, #11099 ),
 .UNSPECIFIED., .F., .T. ) 
 B_SPLINE_CURVE_WITH_KNOTS ( ( 3, 2, 2, 2, 3 ),
 ( 0.5781250000000000000, 0.5859375000000000000, 0.5937500000000000000, 0.6015625000000000000, 0.6093750000000000000 ),
 .UNSPECIFIED. ) 
 CURVE ( )  GEOMETRIC_REPRESENTATION_ITEM ( )  RATIONAL_B_SPLINE_CURVE ( ( 1.000000000000000000, 0.9238795325112867385, 1.000000000000000000, 0.9238795325112867385, 1.000000000000000000, 0.9238795325112867385, 1.000000000000000000, 0.9238795325112867385, 1.000000000000000000 ) ) 
 REPRESENTATION_ITEM ( '' )  );
#23931=VERTEX_POINT ( 'NONE', #10347 ) ;
#23933=CARTESIAN_POINT ( 'NONE',  ( 18.50000000000012790, 1.873492889145011997, 1.873492889144845464 ) ) ;
#23958=CARTESIAN_POINT ( 'NONE',  ( 18.56250000000011013, 2.649519052838358757, -1.097466725451559322 ) ) ;
#23974=CARTESIAN_POINT ( 'NONE',  ( 11.25000000000009237, 1.873492889145011997, -1.873492889144956486 ) ) ;
#23975=CARTESIAN_POINT ( 'NONE',  ( 19.81250000000009237, 0.8284271247463557142, -2.000000000000091926 ) ) ;
#23980=SURFACE_STYLE_USAGE ( .BOTH. , #16655 ) ;
#23996=CARTESIAN_POINT ( 'NONE',  ( 11.08632486540533968, -1.767766952966265404, 1.767766952966376426 ) ) ;
#24033=CARTESIAN_POINT ( 'NONE',  ( 21.56250000000015987, -1.999999999999911626, -0.8284271247462354770 ) ) ;
#24057=CARTESIAN_POINT ( 'NONE',  ( 9.750000000000092371, 1.873492889145011997, 1.873492889144678930 ) ) ;
#24060=( BOUNDED_CURVE ( )  B_SPLINE_CURVE ( 2, ( #4017, #30288, #9097, #9248, #8954, #27814, #8801, #6321, #15750 ),
 .UNSPECIFIED., .F., .F. ) 
 B_SPLINE_CURVE_WITH_KNOTS ( ( 3, 2, 2, 2, 3 ),
 ( 0.4218750000000000000, 0.4296875000000000000, 0.4375000000000000000, 0.4453125000000000000, 0.4531250000000000000 ),
 .UNSPECIFIED. ) 
 CURVE ( )  GEOMETRIC_REPRESENTATION_ITEM ( )  RATIONAL_B_SPLINE_CURVE ( ( 1.000000000000000000, 0.9238795325112867385, 1.000000000000000000, 0.9238795325112867385, 1.000000000000000000, 0.9238795325112867385, 1.000000000000000000, 0.9238795325112867385, 1.000000000000000000 ) ) 
 REPRESENTATION_ITEM ( '' )  );
#24067=ORIENTED_EDGE ( 'NONE', *, *, #5246, .T. ) ;
#24069=CARTESIAN_POINT ( 'NONE',  ( 17.12500000000011369, 1.665334536937734811E-13, -2.649519052838444910 ) ) ;
#24071=AXIS2_PLACEMENT_3D ( 'NONE', #1752, #22966, #25555 ) ;
#24088=AXIS2_PLACEMENT_3D ( 'NONE', #6181, #25058, #20465 ) ;
#24090=EDGE_CURVE ( 'NONE', #21961, #9159, #24060, .T. ) ;
#24096=CARTESIAN_POINT ( 'NONE',  ( 17.62500000000011369, 2.649519052838500421, 0.000000000000000000 ) ) ;
#24115=EDGE_CURVE ( 'NONE', #6843, #22842, #18641, .T. ) ;
#24116=ORIENTED_EDGE ( 'NONE', *, *, #532, .T. ) ;
#24117=CARTESIAN_POINT ( 'NONE',  ( 15.18750000000007105, 0.8284271247462955401, 1.999999999999851674 ) ) ;
#24127=ADVANCED_FACE ( 'NONE', ( #29975 ), #4627, .T. ) ;
#24138=SURFACE_SIDE_STYLE ('',( #21402 ) ) ;
#24144=( BOUNDED_CURVE ( )  B_SPLINE_CURVE ( 2, ( #11734, #16049, #13584, #27801, #20927, #27496, #16350, #4472, #6779 ),
 .UNSPECIFIED., .F., .F. ) 
 B_SPLINE_CURVE_WITH_KNOTS ( ( 3, 2, 2, 2, 3 ),
 ( 0.2968750000000000000, 0.3046875000000000000, 0.3125000000000000000, 0.3203125000000000000, 0.3281250000000000000 ),
 .UNSPECIFIED. ) 
 CURVE ( )  GEOMETRIC_REPRESENTATION_ITEM ( )  RATIONAL_B_SPLINE_CURVE ( ( 1.000000000000000000, 0.9238795325112867385, 1.000000000000000000, 0.9238795325112867385, 1.000000000000000000, 0.9238795325112867385, 1.000000000000000000, 0.9238795325112867385, 1.000000000000000000 ) ) 
 REPRESENTATION_ITEM ( '' )  );
#24150=ADVANCED_FACE ( 'NONE', ( #20323 ), #14207, .T. ) ;
#24174=CARTESIAN_POINT ( 'NONE',  ( 13.81249999999996980, 0.8284271247461753029, -2.000000000000091926 ) ) ;
#24181=CARTESIAN_POINT ( 'NONE',  ( 17.31250000000003908, -0.8284271247461153509, 2.000000000000091926 ) ) ;
#24201=CARTESIAN_POINT ( 'NONE',  ( 23.25000000000004974, 5.551115123125782702E-14, 1.999999999999946265 ) ) ;
#24213=CARTESIAN_POINT ( 'NONE',  ( 19.87500000000008527, -2.649519052838111843, 1.110223024625156540E-13 ) ) ;
#24230=CARTESIAN_POINT ( 'NONE',  ( 24.43750000000014921, -1.999999999999851674, 0.8284271247462354770 ) ) ;
#24236=CARTESIAN_POINT ( 'NONE',  ( 18.62500000000011369, 2.649519052838500421, 0.000000000000000000 ) ) ;
#24248=EDGE_LOOP ( 'NONE', ( #4107, #21775, #7101, #13309 ) ) ;
#24255=ORIENTED_EDGE ( 'NONE', *, *, #27680, .F. ) ;
#24256=CARTESIAN_POINT ( 'NONE',  ( 16.00000000000007105, 2.000000000000223821, -5.551115123125782702E-14 ) ) ;
#24270=B_SPLINE_CURVE_WITH_KNOTS ( 'NONE', 3,
 ( #23486, #2426, #23773, #20716, #9124, #29851, #16381, #15933, #27383, #23275, #4511, #22806, #20964, #25702, #11145, #20493 ),
 .UNSPECIFIED., .F., .F.,
 ( 4, 2, 2, 2, 2, 2, 2, 4 ),
 ( 4.273303003478170257E-15, 0.0005126943745045677188, 0.001025388749004862163, 0.001538083123505156607, 0.002050777498005451269, 0.002563471872505745930, 0.003076166247006041025, 0.004101554996006630781 ),
 .UNSPECIFIED. ) ;
#24272=CARTESIAN_POINT ( 'NONE',  ( 16.96132486540522066, 1.110223024625156540E-13, 2.500000000000002220 ) ) ;
#24278=CARTESIAN_POINT ( 'NONE',  ( 10.75000000000014921, 1.665334536937734811E-13, -2.000000000000168310 ) ) ;
#24311=AXIS2_PLACEMENT_3D ( 'NONE', #25946, #30252, #28240 ) ;
#24320=CARTESIAN_POINT ( 'NONE',  ( 16.06250000000006040, 2.000000000000151879, 0.8284271247461153509 ) ) ;
#24324=CARTESIAN_POINT ( 'NONE',  ( 15.37500000000011013, 2.649519052838500421, -5.551115123125782702E-14 ) ) ;
#24329=DIRECTION ( 'NONE',  ( -1.000000000000000000, -1.665334536937731113E-16, -8.326672684688674053E-17 ) ) ;
#24337=DIRECTION ( 'NONE',  ( -8.326672684688675286E-17, -2.081668171172168821E-17, 1.000000000000000000 ) ) ;
#24345=CARTESIAN_POINT ( 'NONE',  ( 22.00000000000010303, 2.000000000000168310, 0.000000000000000000 ) ) ;
#24365=CARTESIAN_POINT ( 'NONE',  ( 20.31250000000012079, 2.649519052838358757, -1.097466725451559322 ) ) ;
#24372=CARTESIAN_POINT ( 'NONE',  ( 21.10117513459481486, 1.035533905932809473, -2.499999999999904521 ) ) ;
#24390=CARTESIAN_POINT ( 'NONE',  ( 11.03867513459494454, 1.665334536937734811E-13, -2.500000000000113243 ) ) ;
#24401=ORIENTED_EDGE ( 'NONE', *, *, #23182, .F. ) ;
#24406=ORIENTED_EDGE ( 'NONE', *, *, #5141, .F. ) ;
#24412=CARTESIAN_POINT ( 'NONE',  ( 14.68750000000004796, -0.8284271247460552878, -1.999999999999971800 ) ) ;
#24429=ORIENTED_EDGE ( 'NONE', *, *, #11831, .T. ) ;
#24433=CARTESIAN_POINT ( 'NONE',  ( 20.83632486540534856, 1.767766952966487448, 1.767766952966209892 ) ) ;
#24459=CARTESIAN_POINT ( 'NONE',  ( 15.18750000000007105, 0.8284271247462955401, 1.999999999999851674 ) ) ;
#24468=CARTESIAN_POINT ( 'NONE',  ( 15.43750000000009770, -1.999999999999851674, 0.8284271247462354770 ) ) ;
#24473=CARTESIAN_POINT ( 'NONE',  ( 14.25000000000009592, 1.873492889145067508, -1.873492889144956486 ) ) ;
#24481=SURFACE_SIDE_STYLE ('',( #13016 ) ) ;
#24483=CARTESIAN_POINT ( 'NONE',  ( 17.96132486540527751, 1.110223024625156540E-13, 2.499999999999946709 ) ) ;
#24496=CARTESIAN_POINT ( 'NONE',  ( 21.37500000000011724, -1.414213562373090038, 1.414213562373034527 ) ) ;
#24515=CARTESIAN_POINT ( 'NONE',  ( 15.03867513459491967, 1.665334536937734811E-13, -2.500000000000057732 ) ) ;
#24519=EDGE_CURVE ( 'NONE', #22378, #16791, #11360, .T. ) ;
#24522=FACE_OUTER_BOUND ( 'NONE', #21816, .T. ) ;
#24527=CARTESIAN_POINT ( 'NONE',  ( 24.31250000000015277, -0.8284271247461153509, 2.000000000000031530 ) ) ;
#24529=CARTESIAN_POINT ( 'NONE',  ( 23.46132486540525264, 1.110223024625156540E-13, -2.500000000000002220 ) ) ;
#24534=CARTESIAN_POINT ( 'NONE',  ( 16.33632486540528816, -1.767766952966209892, -1.767766952966487448 ) ) ;
#24536=VERTEX_POINT ( 'NONE', #13627 ) ;
#24537=CARTESIAN_POINT ( 'NONE',  ( 15.31250000000012967, -1.097466725451379244, -2.649519052838358757 ) ) ;
#24559=CARTESIAN_POINT ( 'NONE',  ( 15.12500000000000000, 1.414213562373201061, 1.414213562373034527 ) ) ;
#24576=CARTESIAN_POINT ( 'NONE',  ( 24.43750000000014921, 1.097466725451679892, -2.649519052838298805 ) ) ;
#24584=AXIS2_PLACEMENT_3D ( 'NONE', #20248, #3624, #24833 ) ;
#24603=AXIS2_PLACEMENT_3D ( 'NONE', #15509, #15030, #22088 ) ;
#24605=CARTESIAN_POINT ( 'NONE',  ( 10.10117513459485217, 1.035533905932809473, -2.499999999999904521 ) ) ;
#24611=FILL_AREA_STYLE_COLOUR ( '', #17521 ) ;
#24615=CARTESIAN_POINT ( 'NONE',  ( 15.62500000000013856, -1.414213562372979016, -1.414213562373145550 ) ) ;
#24627=CARTESIAN_POINT ( 'NONE',  ( 19.12500000000014211, 1.414213562373256572, 1.414213562373034527 ) ) ;
#24628=ORIENTED_EDGE ( 'NONE', *, *, #6987, .T. ) ;
#24631=CARTESIAN_POINT ( 'NONE',  ( 14.06249999999999645, -1.097466725451439196, -2.649519052838478661 ) ) ;
#24635=CARTESIAN_POINT ( 'NONE',  ( 10.56250000000007461, -1.999999999999971800, -0.8284271247462354770 ) ) ;
#24645=CARTESIAN_POINT ( 'NONE',  ( 19.64882486540529882, 2.500000000000144773, -1.035533905932689347 ) ) ;
#24694=CARTESIAN_POINT ( 'NONE',  ( 14.24999999999998579, -1.873492889144900975, -1.873492889144956486 ) ) ;
#24705=VERTEX_POINT ( 'NONE', #18987 ) ;
#24720=CARTESIAN_POINT ( 'NONE',  ( 16.31250000000011369, -0.8284271247460552878, 1.999999999999971800 ) ) ;
#24737=CARTESIAN_POINT ( 'NONE',  ( 23.50000000000007816, 1.873492889145011997, -1.873492889145067508 ) ) ;
#24739=CARTESIAN_POINT ( 'NONE',  ( 16.46132486540524553, 2.220446049250313081E-13, -2.500000000000002220 ) ) ;
#24789=CARTESIAN_POINT ( 'NONE',  ( 16.56250000000011013, -1.999999999999911626, -0.8284271247462354770 ) ) ;
#24793=ORIENTED_EDGE ( 'NONE', *, *, #18090, .F. ) ;
#24800=CARTESIAN_POINT ( 'NONE',  ( 19.58632486540529172, 1.767766952966542959, -1.767766952966431937 ) ) ;
#24811=CARTESIAN_POINT ( 'NONE',  ( 21.93750000000006395, 2.000000000000212275, -0.8284271247462955401 ) ) ;
#24822=VERTEX_POINT ( 'NONE', #26309 ) ;
#24833=DIRECTION ( 'NONE',  ( -8.326672684688675286E-17, -2.081668171172168821E-17, 1.000000000000000000 ) ) ;
#24845=CARTESIAN_POINT ( 'NONE',  ( 13.93750000000008882, -1.097466725451319070, 2.649519052838238409 ) ) ;
#24869=CARTESIAN_POINT ( 'NONE',  ( 12.12500000000005329, 1.414213562373201061, 1.414213562373034527 ) ) ;
#24883=CARTESIAN_POINT ( 'NONE',  ( 24.62500000000020250, 2.649519052838444910, 0.000000000000000000 ) ) ;
#24888=ORIENTED_EDGE ( 'NONE', *, *, #4778, .T. ) ;
#24893=CARTESIAN_POINT ( 'NONE',  ( 10.00000000000014744, 1.541898448397849286, 1.609913139633878387 ) ) ;
#24918=PLANE ( 'NONE',  #7509 ) ;
#24924=CARTESIAN_POINT ( 'NONE',  ( 13.12500000000016342, 1.414213562373145550, 1.414213562373034527 ) ) ;
#24931=CARTESIAN_POINT ( 'NONE',  ( 14.18749999999996447, 0.8284271247462955401, 2.000000000000031530 ) ) ;
#24934=CARTESIAN_POINT ( 'NONE',  ( 14.81250000000001599, -2.649519052838238409, 1.097466725451559322 ) ) ;
#24953=CARTESIAN_POINT ( 'NONE',  ( 22.25000000000010303, 1.110223024625156540E-13, 1.999999999999946265 ) ) ;
#24969=DIRECTION ( 'NONE',  ( -1.000000000000000000, -1.665334536937731113E-16, 1.526556658859586792E-16 ) ) ;
#24975=AXIS2_PLACEMENT_3D ( 'NONE', #22561, #4252, #15835 ) ;
#24988=CARTESIAN_POINT ( 'NONE',  ( 15.62500000000011013, 2.649519052838389399, -1.110223024625156540E-13 ) ) ;
#25011=CARTESIAN_POINT ( 'NONE',  ( 20.33632486540521001, -1.767766952966209892, -1.767766952966542959 ) ) ;
#25013=CARTESIAN_POINT ( 'NONE',  ( 11.75000000000012079, 1.665334536937734811E-13, -2.000000000000057288 ) ) ;
#25018=CARTESIAN_POINT ( 'NONE',  ( 23.21132486540530948, -2.499999999999891198, -1.110223024625156540E-13 ) ) ;
#25028=DIRECTION ( 'NONE',  ( -8.326672684688675286E-17, -2.081668171172168821E-17, 1.000000000000000000 ) ) ;
#25030=CARTESIAN_POINT ( 'NONE',  ( 23.93750000000009592, -1.097466725451379244, 2.649519052838178457 ) ) ;
#25037=CARTESIAN_POINT ( 'NONE',  ( 10.18750000000014033, 0.8284271247463557142, 2.000000000000031530 ) ) ;
#25040=CARTESIAN_POINT ( 'NONE',  ( 10.00000000000014744, 0.7333107046349622848, 2.235284847858831636 ) ) ;
#25049=CARTESIAN_POINT ( 'NONE',  ( 23.18750000000004619, 0.8284271247462955401, 1.999999999999851674 ) ) ;
#25058=DIRECTION ( 'NONE',  ( -1.000000000000000000, -1.665334536937731113E-16, 1.526556658859586792E-16 ) ) ;
#25059=CARTESIAN_POINT ( 'NONE',  ( 12.22617513459478999, 2.500000000000205169, -1.035533905932869425 ) ) ;
#25063=CARTESIAN_POINT ( 'NONE',  ( 14.03867513459489125, 5.551115123125782702E-14, -2.500000000000057732 ) ) ;
#25067=SURFACE_STYLE_FILL_AREA ( #18051 ) ;
#25078=ORIENTED_EDGE ( 'NONE', *, *, #15702, .T. ) ;
#25079=VECTOR ( 'NONE', #8165, 1000.000000000000114 ) ;
#25082=CARTESIAN_POINT ( 'NONE',  ( 14.68750000000004796, -0.8284271247460553989, -1.999999999999971800 ) ) ;
#25134=CARTESIAN_POINT ( 'NONE',  ( 11.28867513459488947, 2.500000000000002220, 0.000000000000000000 ) ) ;
#25137=CARTESIAN_POINT ( 'NONE',  ( 12.43750000000001776, 1.097466725451679892, -2.649519052838238409 ) ) ;
#25153=( BOUNDED_CURVE ( )  B_SPLINE_CURVE ( 2, ( #28053, #11681, #23180, #6723, #11838, #25769, #29494, #13836, #13995 ),
 .UNSPECIFIED., .F., .T. ) 
 B_SPLINE_CURVE_WITH_KNOTS ( ( 3, 2, 2, 2, 3 ),
 ( 0.3593750000000000000, 0.3671875000000000000, 0.3750000000000000000, 0.3828125000000000000, 0.3906250000000000000 ),
 .UNSPECIFIED. ) 
 CURVE ( )  GEOMETRIC_REPRESENTATION_ITEM ( )  RATIONAL_B_SPLINE_CURVE ( ( 1.000000000000000000, 0.9238795325112867385, 1.000000000000000000, 0.9238795325112867385, 1.000000000000000000, 0.9238795325112867385, 1.000000000000000000, 0.9238795325112867385, 1.000000000000000000 ) ) 
 REPRESENTATION_ITEM ( '' )  );
#25160=CARTESIAN_POINT ( 'NONE',  ( 12.75000000000017764, 1.665334536937734811E-13, -2.000000000000001776 ) ) ;
#25164=DIRECTION ( 'NONE',  ( -1.000000000000000000, -1.665334536937731113E-16, 1.526556658859586792E-16 ) ) ;
#25179=CYLINDRICAL_SURFACE ( 'NONE', #19234, 2.499999999999999112 ) ;
#25195=CARTESIAN_POINT ( 'NONE',  ( 18.78867513459486815, -2.499999999999946709, -5.551115123125782702E-14 ) ) ;
#25197=CARTESIAN_POINT ( 'NONE',  ( 23.87500000000009237, 1.414213562373256572, -1.414213562373145550 ) ) ;
#25226=CARTESIAN_POINT ( 'NONE',  ( 14.25000000000012434, 5.551115123125782702E-14, 2.000000000000001776 ) ) ;
#25248=CARTESIAN_POINT ( 'NONE',  ( 18.37500000000008527, -1.414213562373090038, 1.414213562372867994 ) ) ;
#25257=ORIENTED_EDGE ( 'NONE', *, *, #14025, .T. ) ;
#25258=ORIENTED_EDGE ( 'NONE', *, *, #2146, .T. ) ;
#25279=EDGE_CURVE ( 'NONE', #1574, #30369, #5768, .T. ) ;
#25283=CARTESIAN_POINT ( 'NONE',  ( 11.00000000000003730, -1.873492889144900975, 1.873492889144900975 ) ) ;
#25294=( BOUNDED_CURVE ( )  B_SPLINE_CURVE ( 2, ( #5059, #26261, #16793, #5212, #21678, #2911, #19225, #14489, #7237 ),
 .UNSPECIFIED., .F., .F. ) 
 B_SPLINE_CURVE_WITH_KNOTS ( ( 3, 2, 2, 2, 3 ),
 ( 0.01562500000000000000, 0.02343750000000000000, 0.03125000000000000000, 0.03906250000000000000, 0.04687500000000000000 ),
 .UNSPECIFIED. ) 
 CURVE ( )  GEOMETRIC_REPRESENTATION_ITEM ( )  RATIONAL_B_SPLINE_CURVE ( ( 1.000000000000000000, 0.9238795325112867385, 1.000000000000000000, 0.9238795325112867385, 1.000000000000000000, 0.9238795325112867385, 1.000000000000000000, 0.9238795325112867385, 1.000000000000000000 ) ) 
 REPRESENTATION_ITEM ( '' )  );
#25298=ORIENTED_EDGE ( 'NONE', *, *, #2956, .F. ) ;
#25303=CARTESIAN_POINT ( 'NONE',  ( 21.31250000000007105, 2.649519052838358757, -1.097466725451619718 ) ) ;
#25305=ORIENTED_EDGE ( 'NONE', *, *, #15702, .F. ) ;
#25327=CARTESIAN_POINT ( 'NONE',  ( 20.37500000000017053, 1.665334536937734811E-13, -2.649519052838389399 ) ) ;
#25336=CARTESIAN_POINT ( 'NONE',  ( 17.33632486540525974, -1.767766952966154381, -1.767766952966487448 ) ) ;
#25339=COLOUR_RGB ( '', 0.31764706, 0.68627451, 0.89019608) ;
#25350=CARTESIAN_POINT ( 'NONE',  ( 21.12500000000011724, 1.414213562373201061, 1.414213562373034527 ) ) ;
#25351=DIRECTION ( 'NONE',  ( -1.000000000000000000, -1.665334536937731113E-16, 1.526556658859586792E-16 ) ) ;
#25357=CARTESIAN_POINT ( 'NONE',  ( 12.53867513459494631, 1.110223024625156540E-13, 2.500000000000002220 ) ) ;
#25373=EDGE_LOOP ( 'NONE', ( #1428, #11091, #6702, #760 ) ) ;
#25377=CARTESIAN_POINT ( 'NONE',  ( 13.06249999999998046, 2.000000000000151879, 0.8284271247461152399 ) ) ;
#25381=CARTESIAN_POINT ( 'NONE',  ( 14.46132486540527218, 5.551115123125782702E-14, -2.500000000000057732 ) ) ;
#25385=CARTESIAN_POINT ( 'NONE',  ( 14.62500000000008171, -1.414213562372979016, -1.414213562373145550 ) ) ;
#25389=CARTESIAN_POINT ( 'NONE',  ( 18.41367513459493566, 1.767766952966598470, 1.767766952966320915 ) ) ;
#25406=CARTESIAN_POINT ( 'NONE',  ( 9.999999999999841904, 2.000000000000057288, -4.274358644806852681E-12 ) ) ;
#25410=CARTESIAN_POINT ( 'NONE',  ( 20.87500000000014211, 1.414213562373367594, -1.414213562373145550 ) ) ;
#25416=( NAMED_UNIT ( * ) SI_UNIT ( $, .STERADIAN. ) SOLID_ANGLE_UNIT ( ) );
#25417=CARTESIAN_POINT ( 'NONE',  ( 11.89882486540525797, 1.035533905932749299, 2.499999999999964473 ) ) ;
#25419=ORIENTED_EDGE ( 'NONE', *, *, #27497, .T. ) ;
#25432=( BOUNDED_CURVE ( )  B_SPLINE_CURVE ( 2, ( #12183, #21069, #7515, #26107, #21670, #16926, #19368, #19216, #2755 ),
 .UNSPECIFIED., .F., .T. ) 
 B_SPLINE_CURVE_WITH_KNOTS ( ( 3, 2, 2, 2, 3 ),
 ( 0.7656250000000000000, 0.7734375000000000000, 0.7812500000000000000, 0.7890625000000000000, 0.7968750000000000000 ),
 .UNSPECIFIED. ) 
 CURVE ( )  GEOMETRIC_REPRESENTATION_ITEM ( )  RATIONAL_B_SPLINE_CURVE ( ( 1.000000000000000000, 0.9238795325112867385, 1.000000000000000000, 0.9238795325112867385, 1.000000000000000000, 0.9238795325112867385, 1.000000000000000000, 0.9238795325112867385, 1.000000000000000000 ) ) 
 REPRESENTATION_ITEM ( '' )  );
#25444=CARTESIAN_POINT ( 'NONE',  ( 13.06250000000007105, -2.649519052838178457, 1.097466725451439196 ) ) ;
#25453=VERTEX_POINT ( 'NONE', #10565 ) ;
#25461=CARTESIAN_POINT ( 'NONE',  ( 22.56250000000008527, 1.097466725451679892, 2.649519052838298805 ) ) ;
#25471=CARTESIAN_POINT ( 'NONE',  ( 11.18750000000003908, 0.8284271247462955401, 2.000000000000031530 ) ) ;
#25485=CARTESIAN_POINT ( 'NONE',  ( 19.50000000000009948, 1.873492889145067508, -1.873492889145067508 ) ) ;
#25487=AXIS2_PLACEMENT_3D ( 'NONE', #28780, #24329, #5586 ) ;
#25491=VERTEX_POINT ( 'NONE', #22542 ) ;
#25498=CARTESIAN_POINT ( 'NONE',  ( 10.00000000000012079, -0.6095397823829284967, 2.424553825692621345 ) ) ;
#25501=CARTESIAN_POINT ( 'NONE',  ( 14.53867513459486460, 1.665334536937734811E-13, 2.499999999999835687 ) ) ;
#25509=CARTESIAN_POINT ( 'NONE',  ( 21.68750000000000711, -0.8284271247461753029, -2.000000000000031530 ) ) ;
#25515=CARTESIAN_POINT ( 'NONE',  ( 11.66367513459487526, -1.767766952966265404, 1.767766952966376426 ) ) ;
#25519=DIRECTION ( 'NONE',  ( -1.000000000000000000, -1.665334536937731113E-16, 1.526556658859586792E-16 ) ) ;
#25529=DIRECTION ( 'NONE',  ( -8.326672684688675286E-17, -2.081668171172168821E-17, 1.000000000000000000 ) ) ;
#25531=( NAMED_UNIT ( * ) PLANE_ANGLE_UNIT ( ) SI_UNIT ( $, .RADIAN. ) );
#25542=CARTESIAN_POINT ( 'NONE',  ( 14.27382486540519402, -2.499999999999964473, -1.035533905932749299 ) ) ;
#25546=CARTESIAN_POINT ( 'NONE',  ( 11.75000000000012079, 1.665334536937734811E-13, -2.000000000000057288 ) ) ;
#25547=ORIENTED_EDGE ( 'NONE', *, *, #26734, .F. ) ;
#25549=CARTESIAN_POINT ( 'NONE',  ( 18.35117513459491434, 2.500000000000144773, 1.035533905932689347 ) ) ;
#25554=AXIS2_PLACEMENT_3D ( 'NONE', #21752, #12407, #26474 ) ;
#25555=DIRECTION ( 'NONE',  ( -8.326672684688675286E-17, -2.081668171172168821E-17, 1.000000000000000000 ) ) ;
#25576=CARTESIAN_POINT ( 'NONE',  ( 19.25000000000009948, 1.110223024625156540E-13, 1.999999999999946265 ) ) ;
#25578=DIRECTION ( 'NONE',  ( -1.000000000000000000, -1.665334536937731113E-16, 1.526556658859586792E-16 ) ) ;
#25584=( BOUNDED_CURVE ( )  B_SPLINE_CURVE ( 2, ( #11741, #16204, #25515, #23394, #9242, #21084, #13903, #16055, #21234 ),
 .UNSPECIFIED., .F., .F. ) 
 B_SPLINE_CURVE_WITH_KNOTS ( ( 3, 2, 2, 2, 3 ),
 ( 0.1093750000000000000, 0.1171875000000000000, 0.1250000000000000000, 0.1328125000000000000, 0.1406250000000000000 ),
 .UNSPECIFIED. ) 
 CURVE ( )  GEOMETRIC_REPRESENTATION_ITEM ( )  RATIONAL_B_SPLINE_CURVE ( ( 1.000000000000000000, 0.9238795325112867385, 1.000000000000000000, 0.9238795325112867385, 1.000000000000000000, 0.9238795325112867385, 1.000000000000000000, 0.9238795325112867385, 1.000000000000000000 ) ) 
 REPRESENTATION_ITEM ( '' )  );
#25590=EDGE_CURVE ( 'NONE', #13194, #20580, #7114, .T. ) ;
#25598=AXIS2_PLACEMENT_3D ( 'NONE', #23433, #8838, #18224 ) ;
#25604=CARTESIAN_POINT ( 'NONE',  ( 23.53867513459495342, 1.665334536937734811E-13, 2.499999999999835687 ) ) ;
#25614=CARTESIAN_POINT ( 'NONE',  ( 11.50000000000014921, 1.873492889145067508, -1.873492889145067508 ) ) ;
#25632=CARTESIAN_POINT ( 'NONE',  ( 20.93749999999999289, -2.649519052838238409, -1.097466725451559322 ) ) ;
#25635=EDGE_LOOP ( 'NONE', ( #6917, #17110, #25298, #29001, #25547, #10739, #13314, #25734, #3870, #8104, #24793, #11217, #13532, #14287, #1626, #21953, #6668, #595, #26543, #20638, #4178, #4765, #14899, #9166, #16306, #4909, #23381, #20851, #11881, #1636, #27937, #3160, #19505, #10982, #27711 ) ) ;
#25650=CARTESIAN_POINT ( 'NONE',  ( 20.00000000000018474, -1.873492889144789952, 1.873492889144845464 ) ) ;
#25659=CARTESIAN_POINT ( 'NONE',  ( 19.85117513459492145, -2.499999999999904521, -1.035533905932749299 ) ) ;
#25663=ORIENTED_EDGE ( 'NONE', *, *, #7099, .T. ) ;
#25668=CARTESIAN_POINT ( 'NONE',  ( 9.875000000000078160, -2.649519052838111843, -5.551115123125782702E-14 ) ) ;
#25669=CARTESIAN_POINT ( 'NONE',  ( 19.87500000000017053, 1.414213562373312083, -1.414213562373145550 ) ) ;
#25676=CARTESIAN_POINT ( 'NONE',  ( 12.60117513459493743, -1.035533905932629173, 2.499999999999844569 ) ) ;
#25678=CARTESIAN_POINT ( 'NONE',  ( 24.76476637266523539, -1.543174358739360041, -1.624092575704163544 ) ) ;
#25687=PRESENTATION_STYLE_ASSIGNMENT (( #9872 ) ) ;
#25702=CARTESIAN_POINT ( 'NONE',  ( 10.00000000000015277, 0.08046688801464986496, -2.448371654002133635 ) ) ;
#25705=CARTESIAN_POINT ( 'NONE',  ( 10.50000000000003730, -1.999999999999835243, 0.000000000000000000 ) ) ;
#25720=CARTESIAN_POINT ( 'NONE',  ( 12.96132486540529882, 1.110223024625156540E-13, 2.500000000000002220 ) ) ;
#25734=ORIENTED_EDGE ( 'NONE', *, *, #9012, .F. ) ;
#25736=DIRECTION ( 'NONE',  ( -8.326672684688674053E-17, -2.081668171172168513E-17, 1.000000000000000000 ) ) ;
#25766=CARTESIAN_POINT ( 'NONE',  ( 10.18750000000001954, -2.649519052838298805, -1.097466725451559322 ) ) ;
#25769=CARTESIAN_POINT ( 'NONE',  ( 15.85117513459492145, -2.499999999999964473, -1.035533905932749299 ) ) ;
#25772=CARTESIAN_POINT ( 'NONE',  ( 24.03867513459490013, 1.665334536937734811E-13, -2.500000000000002220 ) ) ;
#25774=CARTESIAN_POINT ( 'NONE',  ( 15.14882486540524198, -2.499999999999904521, 1.035533905932749299 ) ) ;
#25780=ORIENTED_EDGE ( 'NONE', *, *, #11831, .F. ) ;
#25783=CARTESIAN_POINT ( 'NONE',  ( 22.37500000000008882, 2.649519052838555933, -5.551115123125782702E-14 ) ) ;
#25803=CARTESIAN_POINT ( 'NONE',  ( 22.75000000000004974, 1.873492889144956486, 1.873492889144734441 ) ) ;
#25809=DIRECTION ( 'NONE',  ( -1.000000000000000000, -1.665334536937731113E-16, 1.526556658859586792E-16 ) ) ;
#25821=ORIENTED_EDGE ( 'NONE', *, *, #13077, .T. ) ;
#25823=CARTESIAN_POINT ( 'NONE',  ( 11.43750000000009415, 2.649519052838478661, 1.097466725451499370 ) ) ;
#25833=CARTESIAN_POINT ( 'NONE',  ( 24.64495393282636115, -2.193871126647821246, 0.8697444040583612868 ) ) ;
#25850=VERTEX_POINT ( 'NONE', #12666 ) ;
#25885=CARTESIAN_POINT ( 'NONE',  ( 21.81250000000009592, 0.8284271247462955401, -2.000000000000151879 ) ) ;
#25908=CARTESIAN_POINT ( 'NONE',  ( 13.96132486540527218, 1.110223024625156540E-13, 2.499999999999946709 ) ) ;
#25918=CARTESIAN_POINT ( 'NONE',  ( 15.46132486540530238, 1.110223024625156540E-13, -2.500000000000057732 ) ) ;
#25926=CARTESIAN_POINT ( 'NONE',  ( 22.18750000000000000, 1.097466725451559322, -2.649519052838298805 ) ) ;
#25927=ADVANCED_FACE ( 'NONE', ( #20622 ), #11269, .T. ) ;
#25946=CARTESIAN_POINT ( 'NONE',  ( 0.000000000000000000, 0.000000000000000000, 0.000000000000000000 ) ) ;
#25948=CARTESIAN_POINT ( 'NONE',  ( 21.50000000000018474, 1.873492889145067508, -1.873492889145123019 ) ) ;
#25953=CARTESIAN_POINT ( 'NONE',  ( 17.10117513459487171, 1.035533905932929599, -2.499999999999964473 ) ) ;
#25971=CARTESIAN_POINT ( 'NONE',  ( 21.46132486540527751, 5.551115123125782702E-14, -2.500000000000002220 ) ) ;
#25972=CARTESIAN_POINT ( 'NONE',  ( 18.62500000000003197, -1.414213562373034527, -1.414213562373090038 ) ) ;
#25975=DIRECTION ( 'NONE',  ( -1.000000000000000000, -1.665334536937731113E-16, 1.526556658859586792E-16 ) ) ;
#26023=CARTESIAN_POINT ( 'NONE',  ( 16.81250000000007816, 0.8284271247462955401, -2.000000000000091926 ) ) ;
#26026=CARTESIAN_POINT ( 'NONE',  ( 0.000000000000000000, 0.000000000000000000, 0.000000000000000000 ) ) ;
#26035=CARTESIAN_POINT ( 'NONE',  ( 19.31250000000010303, -0.8284271247459350507, 2.000000000000091926 ) ) ;
#26060=CARTESIAN_POINT ( 'NONE',  ( 9.312500000000124345, -1.097466725451499370, -2.649519052838358757 ) ) ;
#26076=CARTESIAN_POINT ( 'NONE',  ( 17.56250000000009592, 1.097466725451619718, 2.649519052838298805 ) ) ;
#26078=ORIENTED_EDGE ( 'NONE', *, *, #11223, .T. ) ;
#26098=CARTESIAN_POINT ( 'NONE',  ( 16.81250000000011013, 1.097466725451619718, 2.649519052838358757 ) ) ;
#26107=CARTESIAN_POINT ( 'NONE',  ( 22.22617513459494987, 2.500000000000084821, -1.035533905932869425 ) ) ;
#26109=ORIENTED_EDGE ( 'NONE', *, *, #12576, .F. ) ;
#26110=CARTESIAN_POINT ( 'NONE',  ( 20.78867513459484329, -2.499999999999891198, -2.220446049250313081E-13 ) ) ;
#26115=CARTESIAN_POINT ( 'NONE',  ( 12.12500000000007994, 1.110223024625156540E-13, -2.649519052838444910 ) ) ;
#26116=CARTESIAN_POINT ( 'NONE',  ( 19.46132486540541606, 1.665334536937734811E-13, -2.500000000000002220 ) ) ;
#26118=CARTESIAN_POINT ( 'NONE',  ( 17.43750000000012790, -1.999999999999851674, 0.8284271247463557142 ) ) ;
#26124=LINE ( 'NONE', #625, #16316 ) ;
#26125=FILL_AREA_STYLE ('',( #9245 ) ) ;
#26127=CARTESIAN_POINT ( 'NONE',  ( 24.59383218691901263, -1.521799583385193166, 1.870049939131334549 ) ) ;
#26133=DIRECTION ( 'NONE',  ( 8.326672684688674053E-17, 2.081668171172168513E-17, -1.000000000000000000 ) ) ;
#26143=STYLED_ITEM ( 'NONE', ( #11903 ), #22780 ) ;
#26178=CARTESIAN_POINT ( 'NONE',  ( 22.68750000000017764, -0.8284271247460553989, -2.000000000000031530 ) ) ;
#26196=CARTESIAN_POINT ( 'NONE',  ( 24.28867513459498184, 2.500000000000057732, -2.220446049250313081E-13 ) ) ;
#26199=CARTESIAN_POINT ( 'NONE',  ( 13.46132486540532724, 1.665334536937734811E-13, -2.500000000000057732 ) ) ;
#26202=CARTESIAN_POINT ( 'NONE',  ( 24.31250000000015632, -0.8284271247461152399, 2.000000000000031530 ) ) ;
#26213=CARTESIAN_POINT ( 'NONE',  ( 19.56250000000012790, 1.097466725451739622, 2.649519052838298805 ) ) ;
#26232=DIRECTION ( 'NONE',  ( -8.326672684688675286E-17, -2.081668171172168821E-17, 1.000000000000000000 ) ) ;
#26240=CARTESIAN_POINT ( 'NONE',  ( 16.21132486540519224, -2.499999999999835687, -1.110223024625156540E-13 ) ) ;
#26242=CARTESIAN_POINT ( 'NONE',  ( 18.12500000000011369, -2.649519052838111843, 0.000000000000000000 ) ) ;
#26261=CARTESIAN_POINT ( 'NONE',  ( 24.39882486540525974, -1.035533905932568999, -2.499999999999964473 ) ) ;
#26262=CARTESIAN_POINT ( 'NONE',  ( 12.31250000000017053, 2.649519052838419153, -1.097466725451619718 ) ) ;
#26264=VERTEX_POINT ( 'NONE', #14593 ) ;
#26265=CARTESIAN_POINT ( 'NONE',  ( 20.87500000000014211, 1.414213562373367594, -1.414213562373145550 ) ) ;
#26272=LINE ( 'NONE', #5222, #4738 ) ;
#26276=DIRECTION ( 'NONE',  ( -8.326672684688675286E-17, -2.081668171172168821E-17, 1.000000000000000000 ) ) ;
#26309=CARTESIAN_POINT ( 'NONE',  ( 20.46132486540533435, 1.110223024625156540E-13, -2.500000000000057732 ) ) ;
#26326=CARTESIAN_POINT ( 'NONE',  ( 20.43750000000014566, -1.999999999999911626, 0.8284271247462354770 ) ) ;
#26328=VERTEX_POINT ( 'NONE', #8233 ) ;
#26332=( BOUNDED_CURVE ( )  B_SPLINE_CURVE ( 2, ( #16340, #4761, #25336, #4311, #13730, #23073, #18470, #6768, #20917 ),
 .UNSPECIFIED., .F., .T. ) 
 B_SPLINE_CURVE_WITH_KNOTS ( ( 3, 2, 2, 2, 3 ),
 ( 0.4531250000000000000, 0.4609375000000000000, 0.4687500000000000000, 0.4765625000000000000, 0.4843750000000000000 ),
 .UNSPECIFIED. ) 
 CURVE ( )  GEOMETRIC_REPRESENTATION_ITEM ( )  RATIONAL_B_SPLINE_CURVE ( ( 1.000000000000000000, 0.9238795325112867385, 1.000000000000000000, 0.9238795325112867385, 1.000000000000000000, 0.9238795325112867385, 1.000000000000000000, 0.9238795325112867385, 1.000000000000000000 ) ) 
 REPRESENTATION_ITEM ( '' )  );
#26346=FACE_OUTER_BOUND ( 'NONE', #18780, .T. ) ;
#26351=CARTESIAN_POINT ( 'NONE',  ( 22.93749999999995737, 1.999999999999971800, -0.8284271247462354770 ) ) ;
#26368=CARTESIAN_POINT ( 'NONE',  ( 19.00000000000018474, -1.873492889144845464, -1.873492889145123019 ) ) ;
#26371=ORIENTED_EDGE ( 'NONE', *, *, #1744, .T. ) ;
#26386=CARTESIAN_POINT ( 'NONE',  ( 23.81250000000003908, 0.8284271247463557142, -2.000000000000151879 ) ) ;
#26399=CARTESIAN_POINT ( 'NONE',  ( 22.89882486540531303, 1.035533905932809473, 2.500000000000024425 ) ) ;
#26413=CARTESIAN_POINT ( 'NONE',  ( 15.43750000000009770, -1.999999999999851674, 0.8284271247462354770 ) ) ;
#26418=( NAMED_UNIT ( * ) SI_UNIT ( $, .STERADIAN. ) SOLID_ANGLE_UNIT ( ) );
#26430=FILL_AREA_STYLE ('',( #17105 ) ) ;
#26435=CARTESIAN_POINT ( 'NONE',  ( 20.71132486540530593, 2.500000000000057732, -1.665334536937734811E-13 ) ) ;
#26440=CARTESIAN_POINT ( 'NONE',  ( 9.812500000000115463, 0.8284271247462955401, -2.000000000000091926 ) ) ;
#26471=CARTESIAN_POINT ( 'NONE',  ( 20.37500000000017053, -1.414213562372979016, 1.414213562373034527 ) ) ;
#26474=DIRECTION ( 'NONE',  ( -8.326672684688675286E-17, -2.081668171172168821E-17, 1.000000000000000000 ) ) ;
#26492=CARTESIAN_POINT ( 'NONE',  ( 24.00000000000013145, 2.000000000000057288, -1.665334536937734811E-13 ) ) ;
#26512=CARTESIAN_POINT ( 'NONE',  ( 18.75000000000012790, -1.873492889144900975, 1.873492889144845464 ) ) ;
#26531=CARTESIAN_POINT ( 'NONE',  ( 24.81250000000012079, 0.8284271247463557142, -2.000000000000091926 ) ) ;
#26532=AXIS2_PLACEMENT_3D ( 'NONE', #8673, #8981, #6054 ) ;
#26538=CARTESIAN_POINT ( 'NONE',  ( 18.75000000000015632, 1.873492889145067508, 1.873492889144734441 ) ) ;
#26543=ORIENTED_EDGE ( 'NONE', *, *, #2146, .F. ) ;
#26548=CARTESIAN_POINT ( 'NONE',  ( 22.71132486540533435, 2.500000000000057732, -1.665334536937734811E-13 ) ) ;
#26562=CARTESIAN_POINT ( 'NONE',  ( 16.18750000000014566, 0.8284271247462955401, 2.000000000000031530 ) ) ;
#26586=AXIS2_PLACEMENT_3D ( 'NONE', #18145, #27457, #29319 ) ;
#26588=DIRECTION ( 'NONE',  ( -1.000000000000000000, -1.665334536937731113E-16, 1.526556658859586792E-16 ) ) ;
#26594=( BOUNDED_CURVE ( )  B_SPLINE_CURVE ( 2, ( #24272, #26870, #1084, #22295, #27030, #5995, #8136, #15570, #24739 ),
 .UNSPECIFIED., .F., .T. ) 
 B_SPLINE_CURVE_WITH_KNOTS ( ( 3, 2, 2, 2, 3 ),
 ( 0.4843750000000000000, 0.4921875000000000000, 0.5000000000000000000, 0.5078125000000000000, 0.5156250000000000000 ),
 .UNSPECIFIED. ) 
 CURVE ( )  GEOMETRIC_REPRESENTATION_ITEM ( )  RATIONAL_B_SPLINE_CURVE ( ( 1.000000000000000000, 0.9238795325112867385, 1.000000000000000000, 0.9238795325112867385, 1.000000000000000000, 0.9238795325112867385, 1.000000000000000000, 0.9238795325112867385, 1.000000000000000000 ) ) 
 REPRESENTATION_ITEM ( '' )  );
#26600=ADVANCED_FACE ( 'NONE', ( #14560 ), #984, .F. ) ;
#26619=CARTESIAN_POINT ( 'NONE',  ( 18.37500000000008527, -1.414213562373090038, 1.414213562372867994 ) ) ;
#26622=CARTESIAN_POINT ( 'NONE',  ( 13.37500000000010836, 2.649519052838444910, -5.551115123125782702E-14 ) ) ;
#26653=CARTESIAN_POINT ( 'NONE',  ( 18.25000000000009948, 1.873492889145123019, -1.873492889144956486 ) ) ;
#26663=CYLINDRICAL_SURFACE ( 'NONE', #24603, 2.499999999999999112 ) ;
#26672=CARTESIAN_POINT ( 'NONE',  ( 23.56250000000009948, -1.999999999999851674, -0.8284271247462354770 ) ) ;
#26677=CARTESIAN_POINT ( 'NONE',  ( 16.39882486540525264, -1.035533905932749299, -2.499999999999964473 ) ) ;
#26679=CARTESIAN_POINT ( 'NONE',  ( 16.31250000000002487, -1.097466725451379244, -2.649519052838419153 ) ) ;
#26697=CARTESIAN_POINT ( 'NONE',  ( 14.87500000000011013, 1.414213562373201061, -1.414213562373090038 ) ) ;
#26699=LINE ( 'NONE', #7975, #23548 ) ;
#26730=CARTESIAN_POINT ( 'NONE',  ( 18.66367513459488237, -1.767766952966154381, 1.767766952966320915 ) ) ;
#26734=EDGE_CURVE ( 'NONE', #1194, #305, #9434, .T. ) ;
#26743=CARTESIAN_POINT ( 'NONE',  ( 10.01999883338032937, -0.3094390903222259404, -2.500000000000104361 ) ) ;
#26750=CARTESIAN_POINT ( 'NONE',  ( 14.12500000000013678, 1.414213562373201061, 1.414213562373034527 ) ) ;
#26760=( BOUNDED_CURVE ( )  B_SPLINE_CURVE ( 2, ( #24483, #1606, #6214, #11010, #20355, #17927, #10860, #15632, #29235 ),
 .UNSPECIFIED., .F., .T. ) 
 B_SPLINE_CURVE_WITH_KNOTS ( ( 3, 2, 2, 2, 3 ),
 ( 0.4218750000000000000, 0.4296875000000000000, 0.4375000000000000000, 0.4453125000000000000, 0.4531250000000000000 ),
 .UNSPECIFIED. ) 
 CURVE ( )  GEOMETRIC_REPRESENTATION_ITEM ( )  RATIONAL_B_SPLINE_CURVE ( ( 1.000000000000000000, 0.9238795325112867385, 1.000000000000000000, 0.9238795325112867385, 1.000000000000000000, 0.9238795325112867385, 1.000000000000000000, 0.9238795325112867385, 1.000000000000000000 ) ) 
 REPRESENTATION_ITEM ( '' )  );
#26762=CARTESIAN_POINT ( 'NONE',  ( 16.68750000000013856, -0.8284271247461753029, -2.000000000000151879 ) ) ;
#26766=CARTESIAN_POINT ( 'NONE',  ( 13.87500000000008171, -2.649519052838111843, 0.000000000000000000 ) ) ;
#26774=FILL_AREA_STYLE ('',( #12862 ) ) ;
#26776=CARTESIAN_POINT ( 'NONE',  ( 19.03867513459492500, 1.110223024625156540E-13, -2.500000000000057732 ) ) ;
#26786=CARTESIAN_POINT ( 'NONE',  ( 21.43750000000007105, -1.999999999999911626, 0.8284271247461753029 ) ) ;
#26790=VERTEX_POINT ( 'NONE', #6514 ) ;
#26794=CARTESIAN_POINT ( 'NONE',  ( 24.97285668889470855, 1.969969495779358759, -0.5495425123464061645 ) ) ;
#26818=CARTESIAN_POINT ( 'NONE',  ( 23.93750000000006750, 2.000000000000151879, -0.8284271247462955401 ) ) ;
#26851=CARTESIAN_POINT ( 'NONE',  ( 15.56250000000003375, -1.999999999999851674, -0.8284271247462354770 ) ) ;
#26854=AXIS2_PLACEMENT_3D ( 'NONE', #7091, #16508, #21391 ) ;
#26869=CARTESIAN_POINT ( 'NONE',  ( 17.66367513459490723, -1.767766952966320915, 1.767766952966431937 ) ) ;
#26870=CARTESIAN_POINT ( 'NONE',  ( 16.89882486540530593, 1.035533905932869425, 2.499999999999904521 ) ) ;
#26876=CARTESIAN_POINT ( 'NONE',  ( 10.87499999999996803, 1.414213562373312083, -1.414213562373145550 ) ) ;
#26884=CARTESIAN_POINT ( 'NONE',  ( 24.81250000000011724, -2.649519052838298805, 1.097466725451559322 ) ) ;
#26919=CARTESIAN_POINT ( 'NONE',  ( 16.12500000000002842, 1.414213562373201061, 1.414213562373034527 ) ) ;
#26925=DIRECTION ( 'NONE',  ( -1.000000000000000000, -1.665334536937731113E-16, 1.526556658859586792E-16 ) ) ;
#26958=EDGE_LOOP ( 'NONE', ( #26371, #24429, #5423, #20420 ) ) ;
#26984=CARTESIAN_POINT ( 'NONE',  ( 13.31250000000006750, -1.097466725451439196, -2.649519052838419153 ) ) ;
#27013=CARTESIAN_POINT ( 'NONE',  ( 16.93750000000001421, 2.000000000000151879, -0.8284271247462354770 ) ) ;
#27030=CARTESIAN_POINT ( 'NONE',  ( 16.71132486540527395, 2.500000000000057732, -5.551115123125782702E-14 ) ) ;
#27070=CARTESIAN_POINT ( 'NONE',  ( 15.75000000000006928, 2.775557561562891351E-13, -2.000000000000057288 ) ) ;
#27079=CARTESIAN_POINT ( 'NONE',  ( 16.75000000000015277, 1.665334536937734811E-13, -2.000000000000001776 ) ) ;
#27084=CARTESIAN_POINT ( 'NONE',  ( 14.93750000000007461, -2.649519052838298805, -1.097466725451559322 ) ) ;
#27099=CARTESIAN_POINT ( 'NONE',  ( 24.45536158780166858, 1.279379774540844616, 2.256154131391882256 ) ) ;
#27126=( BOUNDED_CURVE ( )  B_SPLINE_CURVE ( 2, ( #13192, #1148, #10721, #997, #19608, #28949, #17472, #20061, #12877 ),
 .UNSPECIFIED., .F., .T. ) 
 B_SPLINE_CURVE_WITH_KNOTS ( ( 3, 2, 2, 2, 3 ),
 ( 0.8593750000000000000, 0.8671875000000000000, 0.8750000000000000000, 0.8828125000000000000, 0.8906250000000000000 ),
 .UNSPECIFIED. ) 
 CURVE ( )  GEOMETRIC_REPRESENTATION_ITEM ( )  RATIONAL_B_SPLINE_CURVE ( ( 1.000000000000000000, 0.9238795325112867385, 1.000000000000000000, 0.9238795325112867385, 1.000000000000000000, 0.9238795325112867385, 1.000000000000000000, 0.9238795325112867385, 1.000000000000000000 ) ) 
 REPRESENTATION_ITEM ( '' )  );
#27133=CARTESIAN_POINT ( 'NONE',  ( 10.00000000000012257, -0.6095397823829284967, 2.424553825692621345 ) ) ;
#27140=CARTESIAN_POINT ( 'NONE',  ( 11.53867513459497296, 5.551115123125782702E-14, 2.500000000000002220 ) ) ;
#27143=CARTESIAN_POINT ( 'NONE',  ( 13.25000000000003908, -1.873492889144789952, -1.873492889145123019 ) ) ;
#27158=EDGE_CURVE ( 'NONE', #27870, #29809, #25294, .T. ) ;
#27166=CARTESIAN_POINT ( 'NONE',  ( 12.18750000000008349, 0.8284271247463557142, 1.999999999999851674 ) ) ;
#27181=VERTEX_POINT ( 'NONE', #11892 ) ;
#27184=DIRECTION ( 'NONE',  ( -1.000000000000000000, -1.665334536937731113E-16, 1.526556658859586792E-16 ) ) ;
#27189=CARTESIAN_POINT ( 'NONE',  ( 15.21132486540524553, -2.499999999999780176, -1.110223024625156540E-13 ) ) ;
#27208=DIRECTION ( 'NONE',  ( -8.326672684688675286E-17, -2.081668171172168821E-17, 1.000000000000000000 ) ) ;
#27216=SURFACE_SIDE_STYLE ('',( #17899 ) ) ;
#27231=CARTESIAN_POINT ( 'NONE',  ( 17.62500000000008527, -1.414213562372923505, -1.414213562373145550 ) ) ;
#27234=CARTESIAN_POINT ( 'NONE',  ( 15.06250000000004441, -1.097466725451439196, -2.649519052838419153 ) ) ;
#27269=AXIS2_PLACEMENT_3D ( 'NONE', #27962, #25519, #16358 ) ;
#27280=CARTESIAN_POINT ( 'NONE',  ( 13.10117513459486993, 1.035533905932869425, -2.499999999999904521 ) ) ;
#27286=CARTESIAN_POINT ( 'NONE',  ( 15.68750000000006217, 2.649519052838358757, 1.097466725451379244 ) ) ;
#27290=CARTESIAN_POINT ( 'NONE',  ( 23.60117513459490013, -1.035533905932568999, 2.499999999999844569 ) ) ;
#27295=ORIENTED_EDGE ( 'NONE', *, *, #9505, .F. ) ;
#27296=CONICAL_SURFACE ( 'NONE', #14132, 2.499999999999999112, 0.7853981633974522758 ) ;
#27316=CARTESIAN_POINT ( 'NONE',  ( 12.68750000000013500, -0.8284271247459952248, -1.999999999999911626 ) ) ;
#27318=( BOUNDED_CURVE ( )  B_SPLINE_CURVE ( 2, ( #6996, #25417, #2250, #30036, #20526, #4684, #18398, #30192, #9156 ),
 .UNSPECIFIED., .F., .T. ) 
 B_SPLINE_CURVE_WITH_KNOTS ( ( 3, 2, 2, 2, 3 ),
 ( 0.7968750000000000000, 0.8046875000000000000, 0.8125000000000000000, 0.8203125000000000000, 0.8281250000000000000 ),
 .UNSPECIFIED. ) 
 CURVE ( )  GEOMETRIC_REPRESENTATION_ITEM ( )  RATIONAL_B_SPLINE_CURVE ( ( 1.000000000000000000, 0.9238795325112867385, 1.000000000000000000, 0.9238795325112867385, 1.000000000000000000, 0.9238795325112867385, 1.000000000000000000, 0.9238795325112867385, 1.000000000000000000 ) ) 
 REPRESENTATION_ITEM ( '' )  );
#27331=DIRECTION ( 'NONE',  ( -1.000000000000000000, -1.665334536937731113E-16, 1.526556658859586792E-16 ) ) ;
#27352=CARTESIAN_POINT ( 'NONE',  ( 24.25000000000018829, 1.110223024625156540E-13, 2.000000000000001776 ) ) ;
#27376=CARTESIAN_POINT ( 'NONE',  ( 21.66367513459499605, -1.767766952966265404, 1.767766952966376426 ) ) ;
#27380=CARTESIAN_POINT ( 'NONE',  ( 12.31250000000005151, -0.8284271247461753029, 2.000000000000091926 ) ) ;
#27383=CARTESIAN_POINT ( 'NONE',  ( 10.00000000000015099, 1.428799426191789346, -1.736548481638942487 ) ) ;
#27402=CARTESIAN_POINT ( 'NONE',  ( 19.18750000000004263, 0.8284271247462955401, 2.000000000000031530 ) ) ;
#27404=FACE_OUTER_BOUND ( 'NONE', #1979, .T. ) ;
#27435=CARTESIAN_POINT ( 'NONE',  ( 10.81250000000001243, 1.097466725451619718, 2.649519052838419153 ) ) ;
#27440=AXIS2_PLACEMENT_3D ( 'NONE', #3852, #25351, #6476 ) ;
#27454=EDGE_CURVE ( 'NONE', #8065, #7192, #24144, .T. ) ;
#27457=DIRECTION ( 'NONE',  ( -1.665334536937730866E-16, 1.000000000000000000, 1.432813616264572524E-16 ) ) ;
#27484=( BOUNDED_CURVE ( )  B_SPLINE_CURVE ( 2, ( #30308, #8822, #27376, #27679, #20336, #9116, #13764, #27523, #29687 ),
 .UNSPECIFIED., .F., .T. ) 
 B_SPLINE_CURVE_WITH_KNOTS ( ( 3, 2, 2, 2, 3 ),
 ( 0.7343750000000000000, 0.7421875000000000000, 0.7500000000000000000, 0.7578125000000000000, 0.7656250000000000000 ),
 .UNSPECIFIED. ) 
 CURVE ( )  GEOMETRIC_REPRESENTATION_ITEM ( )  RATIONAL_B_SPLINE_CURVE ( ( 1.000000000000000000, 0.9238795325112867385, 1.000000000000000000, 0.9238795325112867385, 1.000000000000000000, 0.9238795325112867385, 1.000000000000000000, 0.9238795325112867385, 1.000000000000000000 ) ) 
 REPRESENTATION_ITEM ( '' )  );
#27487=CARTESIAN_POINT ( 'NONE',  ( 21.77382486540523843, 2.500000000000084821, 1.035533905932689347 ) ) ;
#27489=AXIS2_PLACEMENT_3D ( 'NONE', #2178, #11581, #16497 ) ;
#27490=( BOUNDED_CURVE ( )  B_SPLINE_CURVE ( 2, ( #16188, #8936, #21219, #13889, #161, #30264, #12027, #18777, #28097 ),
 .UNSPECIFIED., .F., .T. ) 
 B_SPLINE_CURVE_WITH_KNOTS ( ( 3, 2, 2, 2, 3 ),
 ( 0.1406250000000000000, 0.1484375000000000000, 0.1562500000000000000, 0.1640625000000000000, 0.1718750000000000000 ),
 .UNSPECIFIED. ) 
 CURVE ( )  GEOMETRIC_REPRESENTATION_ITEM ( )  RATIONAL_B_SPLINE_CURVE ( ( 1.000000000000000000, 0.9238795325112867385, 1.000000000000000000, 0.9238795325112867385, 1.000000000000000000, 0.9238795325112867385, 1.000000000000000000, 0.9238795325112867385, 1.000000000000000000 ) ) 
 REPRESENTATION_ITEM ( '' )  );
#27492=VERTEX_POINT ( 'NONE', #7083 ) ;
#27496=CARTESIAN_POINT ( 'NONE',  ( 14.85117513459496408, -2.499999999999904521, -1.035533905932809473 ) ) ;
#27497=EDGE_CURVE ( 'NONE', #1194, #19618, #16744, .T. ) ;
#27498=CARTESIAN_POINT ( 'NONE',  ( 21.81250000000009592, 0.8284271247462955401, -2.000000000000151879 ) ) ;
#27518=VECTOR ( 'NONE', #28899, 1000.000000000000000 ) ;
#27521=CARTESIAN_POINT ( 'NONE',  ( 12.75000000000017764, 1.665334536937734811E-13, -2.000000000000001776 ) ) ;
#27523=CARTESIAN_POINT ( 'NONE',  ( 21.97617513459486460, -1.035533905932749299, -2.499999999999964473 ) ) ;
#27527=CARTESIAN_POINT ( 'NONE',  ( 13.93750000000017941, 2.000000000000151879, -0.8284271247462354770 ) ) ;
#27551=CARTESIAN_POINT ( 'NONE',  ( 19.06250000000013500, 2.000000000000091926, 0.8284271247461753029 ) ) ;
#27577=CARTESIAN_POINT ( 'NONE',  ( 23.77382486540529882, 2.500000000000144773, 1.035533905932689347 ) ) ;
#27584=VERTEX_POINT ( 'NONE', #25971 ) ;
#27585=CARTESIAN_POINT ( 'NONE',  ( 12.62500000000010836, 2.649519052838555933, -5.551115123125782702E-14 ) ) ;
#27601=CARTESIAN_POINT ( 'NONE',  ( 22.87500000000008882, -2.649519052838111843, 0.000000000000000000 ) ) ;
#27612=CARTESIAN_POINT ( 'NONE',  ( 11.31250000000006395, -0.8284271247460552878, 2.000000000000031530 ) ) ;
#27628=CARTESIAN_POINT ( 'NONE',  ( 19.87500000000008527, 1.665334536937734811E-13, 2.649519052838278377 ) ) ;
#27643=CARTESIAN_POINT ( 'NONE',  ( 21.89882486540523843, 1.035533905932869425, 2.499999999999844569 ) ) ;
#27652=CARTESIAN_POINT ( 'NONE',  ( 21.31250000000010658, -0.8284271247460552878, 1.999999999999971800 ) ) ;
#27665=CARTESIAN_POINT ( 'NONE',  ( 24.99999999999999289, 1.110223024625156540E-13, -2.220446049250313081E-13 ) ) ;
#27667=ORIENTED_EDGE ( 'NONE', *, *, #20291, .F. ) ;
#27679=CARTESIAN_POINT ( 'NONE',  ( 21.72617513459489658, -2.499999999999904521, 1.035533905932689347 ) ) ;
#27680=EDGE_CURVE ( 'NONE', #16791, #27492, #28610, .T. ) ;
#27682=CARTESIAN_POINT ( 'NONE',  ( 15.06250000000016342, 2.000000000000151879, 0.8284271247461153509 ) ) ;
#27685=CARTESIAN_POINT ( 'NONE',  ( 18.46132486540535922, 1.665334536937734811E-13, -2.500000000000113243 ) ) ;
#27704=CARTESIAN_POINT ( 'NONE',  ( 18.56250000000005329, -1.999999999999971800, -0.8284271247462354770 ) ) ;
#27711=ORIENTED_EDGE ( 'NONE', *, *, #18921, .F. ) ;
#27756=CARTESIAN_POINT ( 'NONE',  ( 21.75000000000010303, -1.873492889144789952, 1.873492889144845464 ) ) ;
#27759=CARTESIAN_POINT ( 'NONE',  ( 10.62500000000013500, -1.414213562372979016, -1.414213562373090038 ) ) ;
#27767=CARTESIAN_POINT ( 'NONE',  ( 13.37500000000019185, -1.414213562372979016, 1.414213562372979016 ) ) ;
#27783=CARTESIAN_POINT ( 'NONE',  ( 21.43750000000001066, 1.097466725451619718, -2.649519052838358757 ) ) ;
#27785=EDGE_CURVE ( 'NONE', #24822, #22378, #1156, .T. ) ;
#27792=CARTESIAN_POINT ( 'NONE',  ( 19.91367513459488237, -1.767766952966154381, -1.767766952966542959 ) ) ;
#27801=CARTESIAN_POINT ( 'NONE',  ( 14.72617513459484506, -2.499999999999904521, 1.035533905932749299 ) ) ;
#27803=CARTESIAN_POINT ( 'NONE',  ( 22.62500000000017408, -1.414213562372867994, -1.414213562373034527 ) ) ;
#27813=CARTESIAN_POINT ( 'NONE',  ( 24.66481880024108619, -2.300353558045364455, 0.4292561541254182877 ) ) ;
#27814=CARTESIAN_POINT ( 'NONE',  ( 16.85117513459481842, -2.499999999999904521, -1.035533905932749299 ) ) ;
#27834=CARTESIAN_POINT ( 'NONE',  ( 14.08632486540523132, -1.767766952966320915, 1.767766952966431937 ) ) ;
#27838=CARTESIAN_POINT ( 'NONE',  ( 13.25000000000017764, 5.551115123125782702E-14, 1.999999999999890754 ) ) ;
#27841=CARTESIAN_POINT ( 'NONE',  ( 18.28867513459494987, 2.500000000000113243, -5.551115123125782702E-14 ) ) ;
#27862=LINE ( 'NONE', #20987, #2243 ) ;
#27865=CARTESIAN_POINT ( 'NONE',  ( 20.37500000000017053, -1.414213562372979016, 1.414213562373034527 ) ) ;
#27870=VERTEX_POINT ( 'NONE', #20735 ) ;
#27876=ORIENTED_EDGE ( 'NONE', *, *, #473, .T. ) ;
#27897=CARTESIAN_POINT ( 'NONE',  ( 13.18750000000012967, -2.649519052838238409, -1.097466725451559322 ) ) ;
#27909=CARTESIAN_POINT ( 'NONE',  ( 23.12500000000011724, 1.665334536937734811E-13, -2.649519052838333888 ) ) ;
#27916=FACE_OUTER_BOUND ( 'NONE', #15955, .T. ) ;
#27918=CARTESIAN_POINT ( 'NONE',  ( 10.68750000000004263, -0.8284271247460552878, -1.999999999999971800 ) ) ;
#27933=CARTESIAN_POINT ( 'NONE',  ( 20.62500000000011369, 2.649519052838500421, -5.551115123125782702E-14 ) ) ;
#27937=ORIENTED_EDGE ( 'NONE', *, *, #30127, .F. ) ;
#27940=LINE ( 'NONE', #20914, #15270 ) ;
#27949=CARTESIAN_POINT ( 'NONE',  ( 10.62500000000010658, 1.665334536937734811E-13, 2.649519052838333888 ) ) ;
#27952=CARTESIAN_POINT ( 'NONE',  ( 22.75000000000015987, 1.110223024625156540E-13, -2.000000000000168310 ) ) ;
#27956=ADVANCED_FACE ( 'NONE', ( #27916 ), #6893, .T. ) ;
#27962=CARTESIAN_POINT ( 'NONE',  ( 0.000000000000000000, 0.000000000000000000, 0.000000000000000000 ) ) ;
#28014=CARTESIAN_POINT ( 'NONE',  ( 21.12500000000011724, 1.414213562373201061, 1.414213562373034527 ) ) ;
#28021=FILL_AREA_STYLE_COLOUR ( '', #25339 ) ;
#28032=ADVANCED_FACE ( 'NONE', ( #10232 ), #3132, .T. ) ;
#28038=EDGE_LOOP ( 'NONE', ( #14410, #17847, #13810, #10338 ) ) ;
#28041=CARTESIAN_POINT ( 'NONE',  ( 23.10117513459496763, 1.035533905932809473, -2.499999999999904521 ) ) ;
#28046=CARTESIAN_POINT ( 'NONE',  ( 21.08632486540515316, -1.767766952966154381, 1.767766952966376426 ) ) ;
#28051=CARTESIAN_POINT ( 'NONE',  ( 11.06249999999994671, -2.649519052838298805, 1.097466725451499370 ) ) ;
#28053=CARTESIAN_POINT ( 'NONE',  ( 15.53867513459491967, 1.110223024625156540E-13, 2.499999999999835687 ) ) ;
#28062=EDGE_LOOP ( 'NONE', ( #17000, #7326, #25663, #7916 ) ) ;
#28067=CARTESIAN_POINT ( 'NONE',  ( 22.74999999999999289, -1.873492889144900975, 1.873492889144845464 ) ) ;
#28088=CARTESIAN_POINT ( 'NONE',  ( 21.00000000000012790, -1.873492889144789952, 1.873492889144845464 ) ) ;
#28097=CARTESIAN_POINT ( 'NONE',  ( 21.96132486540530593, 1.665334536937734811E-13, 2.499999999999946709 ) ) ;
#28103=CARTESIAN_POINT ( 'NONE',  ( 20.53867513459481486, 0.000000000000000000, 2.500000000000002220 ) ) ;
#28108=CARTESIAN_POINT ( 'NONE',  ( 11.62500000000007994, 1.110223024625156540E-13, 2.649519052838167354 ) ) ;
#28110=CARTESIAN_POINT ( 'NONE',  ( 18.25000000000009948, 1.110223024625156540E-13, 1.999999999999946265 ) ) ;
#28112=B_SPLINE_CURVE_WITH_KNOTS ( 'NONE', 3,
 ( #8064, #11025, #3913, #17481, #3452, #10556, #22376, #5609, #20070, #13342, #15016, #26794, #5759, #29416 ),
 .UNSPECIFIED., .F., .F.,
 ( 4, 2, 2, 2, 2, 2, 4 ),
 ( 0.007875088219727693212, 0.008688851078647757617, 0.009095732508107790687, 0.009502613937567822022, 0.009909495367027855092, 0.01031637679648788816, 0.01113013965540795257 ),
 .UNSPECIFIED. ) ;
#28135=CARTESIAN_POINT ( 'NONE',  ( 11.43750000000003197, -1.999999999999911626, 0.8284271247462955401 ) ) ;
#28177=CARTESIAN_POINT ( 'NONE',  ( 20.62500000000014211, -1.414213562372979016, -1.414213562373145550 ) ) ;
#28192=EDGE_CURVE ( 'NONE', #13355, #18612, #12355, .T. ) ;
#28201=CARTESIAN_POINT ( 'NONE',  ( 23.68750000000013500, -0.8284271247461152399, -1.999999999999911626 ) ) ;
#28210=CARTESIAN_POINT ( 'NONE',  ( 0.000000000000000000, 0.000000000000000000, 0.000000000000000000 ) ) ;
#28221=CARTESIAN_POINT ( 'NONE',  ( 23.43750000000010303, 2.649519052838419153, 1.097466725451499370 ) ) ;
#28230=DIRECTION ( 'NONE',  ( 0.000000000000000000, -2.081668171172248940E-17, 1.000000000000000000 ) ) ;
#28240=DIRECTION ( 'NONE',  ( -8.326672684688675286E-17, -2.081668171172168821E-17, 1.000000000000000000 ) ) ;
#28242=CARTESIAN_POINT ( 'NONE',  ( 19.93750000000012434, -1.097466725451379244, 2.649519052838238409 ) ) ;
#28248=ORIENTED_EDGE ( 'NONE', *, *, #24090, .T. ) ;
#28262=CARTESIAN_POINT ( 'NONE',  ( 18.81250000000011013, 0.8284271247462354770, -2.000000000000091926 ) ) ;
#28299=STYLED_ITEM ( 'NONE', ( #6841 ), #17780 ) ;
#28325=CARTESIAN_POINT ( 'NONE',  ( 14.52382486540527928, 1.035533905932809473, -2.499999999999904521 ) ) ;
#28329=CARTESIAN_POINT ( 'NONE',  ( 20.93750000000008171, 2.000000000000212275, -0.8284271247463557142 ) ) ;
#28352=CARTESIAN_POINT ( 'NONE',  ( 23.93750000000006750, 2.000000000000151879, -0.8284271247462955401 ) ) ;
#28353=UNCERTAINTY_MEASURE_WITH_UNIT (LENGTH_MEASURE( 1.000000000000000082E-05 ), #21236, 'distance_accuracy_value', 'NONE');
#28365=CARTESIAN_POINT ( 'NONE',  ( 18.18750000000008882, 1.097466725451619718, -2.649519052838358757 ) ) ;
#28386=CARTESIAN_POINT ( 'NONE',  ( 10.00000000000012079, -0.6095397823829284967, 2.424553825692621345 ) ) ;
#28388=CARTESIAN_POINT ( 'NONE',  ( 17.18750000000004263, -2.649519052838178457, -1.097466725451619718 ) ) ;
#28397=ORIENTED_EDGE ( 'NONE', *, *, #2756, .T. ) ;
#28409=CARTESIAN_POINT ( 'NONE',  ( 20.00000000000004619, 2.000000000000057288, -5.551115123125782702E-14 ) ) ;
#28417=DIRECTION ( 'NONE',  ( 1.526556658859587038E-16, -2.081668171172187002E-17, 1.000000000000000000 ) ) ;
#28418=CARTESIAN_POINT ( 'NONE',  ( 24.56825942016106623, -1.021360606787547365, 2.212070257063908585 ) ) ;
#28427=CARTESIAN_POINT ( 'NONE',  ( 1.110223024625156540E-13, 6.000000000000172307, 0.000000000000000000 ) ) ;
#28430=DIRECTION ( 'NONE',  ( 0.000000000000000000, -2.755434769241566700E-14, 1.000000000000000000 ) ) ;
#28447=UNCERTAINTY_MEASURE_WITH_UNIT (LENGTH_MEASURE( 1.000000000000000082E-05 ), #19456, 'distance_accuracy_value', 'NONE');
#28448=CARTESIAN_POINT ( 'NONE',  ( 9.999999999999841904, 2.000000000000057288, -4.274358644806852681E-12 ) ) ;
#28467=CARTESIAN_POINT ( 'NONE',  ( 17.93750000000012434, 2.000000000000091926, -0.8284271247463557142 ) ) ;
#28481=CARTESIAN_POINT ( 'NONE',  ( 19.56250000000009592, -1.999999999999911626, -0.8284271247461753029 ) ) ;
#28499=CARTESIAN_POINT ( 'NONE',  ( 24.03867513459490013, 1.665334536937734811E-13, -2.500000000000002220 ) ) ;
#28506=ORIENTED_EDGE ( 'NONE', *, *, #1744, .F. ) ;
#28513=CARTESIAN_POINT ( 'NONE',  ( 16.93750000000004619, -2.649519052838238409, -1.097466725451559322 ) ) ;
#28521=VERTEX_POINT ( 'NONE', #19563 ) ;
#28533=CARTESIAN_POINT ( 'NONE',  ( 16.27382486540525619, -2.499999999999964473, -1.035533905932749299 ) ) ;
#28535=CARTESIAN_POINT ( 'NONE',  ( 17.50000000000007105, 1.873492889145123019, -1.873492889145011997 ) ) ;
#28555=CARTESIAN_POINT ( 'NONE',  ( 11.37499999999999645, 2.649519052838500421, -5.551115123125782702E-14 ) ) ;
#28558=CARTESIAN_POINT ( 'NONE',  ( 18.12500000000000355, 1.414213562373090038, 1.414213562373090038 ) ) ;
#28607=CARTESIAN_POINT ( 'NONE',  ( 0.000000000000000000, 0.000000000000000000, 0.000000000000000000 ) ) ;
#28608=CARTESIAN_POINT ( 'NONE',  ( 18.00000000000012790, 2.000000000000112799, 0.000000000000000000 ) ) ;
#28610=( BOUNDED_CURVE ( )  B_SPLINE_CURVE ( 2, ( #26116, #23828, #14627, #5507, #14915, #2764, #3202, #12192, #21533 ),
 .UNSPECIFIED., .F., .F. ) 
 B_SPLINE_CURVE_WITH_KNOTS ( ( 3, 2, 2, 2, 3 ),
 ( 0.3281250000000000000, 0.3359375000000000000, 0.3437500000000000000, 0.3515625000000000000, 0.3593750000000000000 ),
 .UNSPECIFIED. ) 
 CURVE ( )  GEOMETRIC_REPRESENTATION_ITEM ( )  RATIONAL_B_SPLINE_CURVE ( ( 1.000000000000000000, 0.9238795325112867385, 1.000000000000000000, 0.9238795325112867385, 1.000000000000000000, 0.9238795325112867385, 1.000000000000000000, 0.9238795325112867385, 1.000000000000000000 ) ) 
 REPRESENTATION_ITEM ( '' )  );
#28618=CARTESIAN_POINT ( 'NONE',  ( 22.12500000000006040, 1.414213562373145550, 1.414213562373201061 ) ) ;
#28632=EDGE_CURVE ( 'NONE', #23931, #18612, #11890, .T. ) ;
#28642=CARTESIAN_POINT ( 'NONE',  ( 23.62500000000000711, -1.414213562372923505, -1.414213562373145550 ) ) ;
#28655=CARTESIAN_POINT ( 'NONE',  ( 18.31250000000011724, 2.649519052838478661, -1.097466725451679892 ) ) ;
#28681=CARTESIAN_POINT ( 'NONE',  ( 18.00000000000007105, -1.873492889144845464, 1.873492889144900975 ) ) ;
#28692=ORIENTED_EDGE ( 'NONE', *, *, #28632, .T. ) ;
#28697=AXIS2_PLACEMENT_3D ( 'NONE', #2411, #23473, #21162 ) ;
#28704=CARTESIAN_POINT ( 'NONE',  ( 19.56250000000009948, -1.999999999999911626, -0.8284271247461753029 ) ) ;
#28707=DIRECTION ( 'NONE',  ( 0.000000000000000000, -2.081668171172247091E-17, 1.000000000000000000 ) ) ;
#28710=CARTESIAN_POINT ( 'NONE',  ( 15.47617513459492500, 1.035533905932809473, 2.499999999999844569 ) ) ;
#28729=CARTESIAN_POINT ( 'NONE',  ( 20.64882486540534501, 2.500000000000084821, -1.035533905932869425 ) ) ;
#28762=CARTESIAN_POINT ( 'NONE',  ( 17.18750000000013145, 0.8284271247463557142, 1.999999999999971800 ) ) ;
#28765=VERTEX_POINT ( 'NONE', #9243 ) ;
#28770=CARTESIAN_POINT ( 'NONE',  ( 21.75000000000007461, 2.220446049250313081E-13, -2.000000000000001776 ) ) ;
#28780=CARTESIAN_POINT ( 'NONE',  ( 24.99999999999999289, 1.110223024625156540E-13, -2.220446049250313081E-13 ) ) ;
#28794=FACE_OUTER_BOUND ( 'NONE', #14477, .T. ) ;
#28796=CARTESIAN_POINT ( 'NONE',  ( 25.00000000000013500, 2.000000000000279332, -5.551115123125782702E-14 ) ) ;
#28800=CARTESIAN_POINT ( 'NONE',  ( 20.22617513459488592, 2.500000000000205169, -1.035533905932929599 ) ) ;
#28809=EDGE_CURVE ( 'NONE', #19802, #30369, #9720, .T. ) ;
#28811=CARTESIAN_POINT ( 'NONE',  ( 19.18750000000007461, 1.097466725451619718, -2.649519052838298805 ) ) ;
#28821=EDGE_CURVE ( 'NONE', #2749, #23806, #7540, .T. ) ;
#28829=CARTESIAN_POINT ( 'NONE',  ( 24.50000000000015987, -1.999999999999835243, -5.551115123125782702E-14 ) ) ;
#28856=CARTESIAN_POINT ( 'NONE',  ( 10.75000000000014921, 1.665334536937734811E-13, -2.000000000000168310 ) ) ;
#28861=CARTESIAN_POINT ( 'NONE',  ( 17.37500000000011369, -1.414213562372979016, 1.414213562373034527 ) ) ;
#28879=SURFACE_STYLE_USAGE ( .BOTH. , #24138 ) ;
#28890=FACE_OUTER_BOUND ( 'NONE', #18200, .T. ) ;
#28899=DIRECTION ( 'NONE',  ( -1.000000000000000000, -1.665334536937731113E-16, 1.526556658859586792E-16 ) ) ;
#28913=EDGE_CURVE ( 'NONE', #23806, #29780, #26124, .T. ) ;
#28925=CARTESIAN_POINT ( 'NONE',  ( 15.68750000000012434, -0.8284271247459350507, -2.000000000000031530 ) ) ;
#28931=CARTESIAN_POINT ( 'NONE',  ( 21.53867513459484329, 0.000000000000000000, 2.500000000000002220 ) ) ;
#28947=CARTESIAN_POINT ( 'NONE',  ( 22.62500000000017408, -1.414213562372867994, -1.414213562373034527 ) ) ;
#28949=CARTESIAN_POINT ( 'NONE',  ( 10.64882486540527395, 2.500000000000144773, -1.035533905932929599 ) ) ;
#28951=CARTESIAN_POINT ( 'NONE',  ( 20.03867513459486815, 1.665334536937734811E-13, -2.500000000000057732 ) ) ;
#28962=ORIENTED_EDGE ( 'NONE', *, *, #1817, .T. ) ;
#28964=CARTESIAN_POINT ( 'NONE',  ( 19.75000000000009948, -1.873492889144789952, 1.873492889144900975 ) ) ;
#28971=ORIENTED_EDGE ( 'NONE', *, *, #16238, .T. ) ;
#28973=CARTESIAN_POINT ( 'NONE',  ( 22.78867513459492500, -2.499999999999891198, -5.551115123125782702E-14 ) ) ;
#28987=CARTESIAN_POINT ( 'NONE',  ( 17.68750000000000355, 2.649519052838298805, 1.097466725451439196 ) ) ;
#29001=ORIENTED_EDGE ( 'NONE', *, *, #13341, .F. ) ;
#29006=CARTESIAN_POINT ( 'NONE',  ( 20.02382486540529172, -1.035533905932568999, 2.499999999999844569 ) ) ;
#29008=CARTESIAN_POINT ( 'NONE',  ( 15.81250000000000178, 0.8284271247462354770, -2.000000000000151879 ) ) ;
#29035=CARTESIAN_POINT ( 'NONE',  ( 10.56250000000007461, -1.999999999999971800, -0.8284271247462354770 ) ) ;
#29037=CARTESIAN_POINT ( 'NONE',  ( 11.27382486540526685, -2.499999999999904521, -1.035533905932749299 ) ) ;
#29041=CARTESIAN_POINT ( 'NONE',  ( 9.937500000000083489, 2.000000000000151879, -0.8284271247463557142 ) ) ;
#29056=LINE ( 'NONE', #12827, #25079 ) ;
#29066=CARTESIAN_POINT ( 'NONE',  ( 14.37500000000016520, -1.414213562373034527, 1.414213562372979016 ) ) ;
#29074=CARTESIAN_POINT ( 'NONE',  ( 16.81250000000007816, 0.8284271247462955401, -2.000000000000091926 ) ) ;
#29078=CARTESIAN_POINT ( 'NONE',  ( 14.87500000000011013, -2.649519052838111843, 0.000000000000000000 ) ) ;
#29096=CARTESIAN_POINT ( 'NONE',  ( 18.46132486540535922, 1.665334536937734811E-13, -2.500000000000113243 ) ) ;
#29103=DIRECTION ( 'NONE',  ( -8.326672684688675286E-17, -2.081668171172168821E-17, 1.000000000000000000 ) ) ;
#29107=CLOSED_SHELL ( 'NONE', ( #2752, #4215, #13283, #12573, #13809, #25927, #6717, #21709, #8881, #19116, #27956, #11114, #29557, #24150, #10609, #30307, #11551, #16018, #1225, #10335, #19149, #3501, #5578, #24127, #16166, #17592, #14524, #28032, #16228, #19419, #2256, #14717, #22075, #21644, #26600, #14264, #17780, #22780, #6118, #17287 ) ) ;
#29108=ORIENTED_EDGE ( 'NONE', *, *, #14651, .F. ) ;
#29110=CARTESIAN_POINT ( 'NONE',  ( 16.75000000000015277, -1.873492889144789952, 1.873492889144956486 ) ) ;
#29116=CARTESIAN_POINT ( 'NONE',  ( 21.41367513459496763, 1.767766952966487448, 1.767766952966376426 ) ) ;
#29129=CARTESIAN_POINT ( 'NONE',  ( 24.18750000000015277, 0.8284271247463557142, 2.000000000000031530 ) ) ;
#29136=CARTESIAN_POINT ( 'NONE',  ( 16.06250000000006040, -2.649519052838238409, 1.097466725451379244 ) ) ;
#29156=CARTESIAN_POINT ( 'NONE',  ( 13.87500000000011013, 1.414213562373312083, -1.414213562373145550 ) ) ;
#29188=CARTESIAN_POINT ( 'NONE',  ( 9.875000000000023093, 1.414213562373201061, -1.414213562373090038 ) ) ;
#29199=LINE ( 'NONE', #8160, #27518 ) ;
#29212=CARTESIAN_POINT ( 'NONE',  ( 16.31250000000011369, -0.8284271247460552878, 1.999999999999971800 ) ) ;
#29222=CARTESIAN_POINT ( 'NONE',  ( 16.37500000000008527, -1.414213562373090038, 1.414213562373034527 ) ) ;
#29223=ORIENTED_EDGE ( 'NONE', *, *, #26734, .T. ) ;
#29227=CARTESIAN_POINT ( 'NONE',  ( 13.25000000000015099, 1.873492889145123019, -1.873492889144956486 ) ) ;
#29230=CARTESIAN_POINT ( 'NONE',  ( 0.000000000000000000, 0.000000000000000000, 0.000000000000000000 ) ) ;
#29235=CARTESIAN_POINT ( 'NONE',  ( 17.46132486540527395, 5.551115123125782702E-14, -2.500000000000002220 ) ) ;
#29240=STYLED_ITEM ( 'NONE', ( #22639 ), #4002 ) ;
#29241=CARTESIAN_POINT ( 'NONE',  ( 19.46132486540541606, 1.665334536937734811E-13, -2.500000000000002220 ) ) ;
#29249=CARTESIAN_POINT ( 'NONE',  ( 21.31250000000010658, -0.8284271247460552878, 1.999999999999971800 ) ) ;
#29275=CARTESIAN_POINT ( 'NONE',  ( 0.000000000000000000, 0.000000000000000000, 0.000000000000000000 ) ) ;
#29285=( BOUNDED_CURVE ( )  B_SPLINE_CURVE ( 2, ( #28103, #14044, #9082, #6773, #26110, #166, #2329, #23382, #14485 ),
 .UNSPECIFIED., .F., .F. ) 
 B_SPLINE_CURVE_WITH_KNOTS ( ( 3, 2, 2, 2, 3 ),
 ( 0.6718750000000000000, 0.6796875000000000000, 0.6875000000000000000, 0.6953125000000000000, 0.7031250000000000000 ),
 .UNSPECIFIED. ) 
 CURVE ( )  GEOMETRIC_REPRESENTATION_ITEM ( )  RATIONAL_B_SPLINE_CURVE ( ( 1.000000000000000000, 0.9238795325112867385, 1.000000000000000000, 0.9238795325112867385, 1.000000000000000000, 0.9238795325112867385, 1.000000000000000000, 0.9238795325112867385, 1.000000000000000000 ) ) 
 REPRESENTATION_ITEM ( '' )  );
#29291=CARTESIAN_POINT ( 'NONE',  ( 13.37500000000013678, 1.665334536937734811E-13, -2.649519052838444910 ) ) ;
#29304=CARTESIAN_POINT ( 'NONE',  ( 24.57756289884257939, 1.057017408232165723, -2.193898053493716471 ) ) ;
#29309=EDGE_CURVE ( 'NONE', #17836, #19610, #23652, .T. ) ;
#29319=DIRECTION ( 'NONE',  ( -1.000000000000000000, -1.665334536937723717E-16, 0.000000000000000000 ) ) ;
#29333=CARTESIAN_POINT ( 'NONE',  ( 23.68750000000009948, 2.649519052838538613, 1.097466725451559322 ) ) ;
#29362=DIRECTION ( 'NONE',  ( -1.000000000000000000, -1.665334536937731113E-16, 1.526556658859586792E-16 ) ) ;
#29372=CARTESIAN_POINT ( 'NONE',  ( 15.06250000000016165, 2.000000000000151879, 0.8284271247461152399 ) ) ;
#29383=CARTESIAN_POINT ( 'NONE',  ( 17.37500000000011369, -1.414213562372979016, 1.414213562373034527 ) ) ;
#29396=CARTESIAN_POINT ( 'NONE',  ( 19.46132486540541606, 1.665334536937734811E-13, -2.500000000000002220 ) ) ;
#29400=CARTESIAN_POINT ( 'NONE',  ( 24.49999999999999289, 0.6095397824026904665, 2.424553825690067388 ) ) ;
#29416=CARTESIAN_POINT ( 'NONE',  ( 25.00000000000013500, 2.000000000000279332, -5.551115123125782702E-14 ) ) ;
#29417=VERTEX_POINT ( 'NONE', #7784 ) ;
#29426=CARTESIAN_POINT ( 'NONE',  ( 21.35117513459487171, 2.500000000000024425, 1.035533905932629173 ) ) ;
#29434=CARTESIAN_POINT ( 'NONE',  ( 10.08632486540522777, -1.767766952966209892, 1.767766952966431937 ) ) ;
#29438=CARTESIAN_POINT ( 'NONE',  ( 13.53867513459486283, 1.110223024625156540E-13, 2.499999999999946709 ) ) ;
#29443=CARTESIAN_POINT ( 'NONE',  ( 16.12500000000019540, -2.649519052838111843, -5.551115123125782702E-14 ) ) ;
#29472=CARTESIAN_POINT ( 'NONE',  ( 15.62500000000013856, -1.414213562372979016, -1.414213562373145550 ) ) ;
#29492=CARTESIAN_POINT ( 'NONE',  ( 17.91367513459496408, -1.767766952966209892, -1.767766952966542959 ) ) ;
#29494=CARTESIAN_POINT ( 'NONE',  ( 15.91367513459493388, -1.767766952966320915, -1.767766952966542959 ) ) ;
#29497=ORIENTED_EDGE ( 'NONE', *, *, #30127, .T. ) ;
#29508=CARTESIAN_POINT ( 'NONE',  ( 21.71132486540530593, 2.500000000000002220, -1.665334536937734811E-13 ) ) ;
#29533=( BOUNDED_CURVE ( )  B_SPLINE_CURVE ( 2, ( #21049, #9364, #6285, #15708, #25018, #18451, #13397, #6437, #6749 ),
 .UNSPECIFIED., .F., .F. ) 
 B_SPLINE_CURVE_WITH_KNOTS ( ( 3, 2, 2, 2, 3 ),
 ( 0.07812500000000000000, 0.08593750000000000000, 0.09375000000000000000, 0.1015625000000000000, 0.1093750000000000000 ),
 .UNSPECIFIED. ) 
 CURVE ( )  GEOMETRIC_REPRESENTATION_ITEM ( )  RATIONAL_B_SPLINE_CURVE ( ( 1.000000000000000000, 0.9238795325112867385, 1.000000000000000000, 0.9238795325112867385, 1.000000000000000000, 0.9238795325112867385, 1.000000000000000000, 0.9238795325112867385, 1.000000000000000000 ) ) 
 REPRESENTATION_ITEM ( '' )  );
#29541=CARTESIAN_POINT ( 'NONE',  ( 14.81250000000010658, 0.8284271247463557142, -2.000000000000031530 ) ) ;
#29550=CARTESIAN_POINT ( 'NONE',  ( 17.75000000000015632, 1.110223024625156540E-13, -2.000000000000001776 ) ) ;
#29553=CARTESIAN_POINT ( 'NONE',  ( 15.18750000000004086, 1.097466725451679892, -2.649519052838238409 ) ) ;
#29557=ADVANCED_FACE ( 'NONE', ( #24522 ), #15032, .T. ) ;
#29569=VECTOR ( 'NONE', #18389, 1000.000000000000000 ) ;
#29586=CARTESIAN_POINT ( 'NONE',  ( 16.25000000000009948, 1.873492889145123019, -1.873492889145011997 ) ) ;
#29607=CARTESIAN_POINT ( 'NONE',  ( 14.31249999999993072, -1.097466725451559322, -2.649519052838358757 ) ) ;
#29629=CARTESIAN_POINT ( 'NONE',  ( 12.31250000000004974, -0.8284271247461753029, 2.000000000000091926 ) ) ;
#29643=CARTESIAN_POINT ( 'NONE',  ( 23.18750000000004619, -2.649519052838238409, -1.097466725451559322 ) ) ;
#29649=CARTESIAN_POINT ( 'NONE',  ( 9.562500000000090594, -1.999999999999851674, -0.8284271247462354770 ) ) ;
#29662=CARTESIAN_POINT ( 'NONE',  ( 23.68750000000013500, -0.8284271247461152399, -1.999999999999911626 ) ) ;
#29669=CARTESIAN_POINT ( 'NONE',  ( 23.96132486540522422, 5.551115123125782702E-14, 2.500000000000002220 ) ) ;
#29672=DIRECTION ( 'NONE',  ( -1.000000000000000000, -1.665334536937731113E-16, 1.526556658859586792E-16 ) ) ;
#29675=CARTESIAN_POINT ( 'NONE',  ( 16.10117513459491789, 1.035533905932869425, -2.499999999999904521 ) ) ;
#29687=CARTESIAN_POINT ( 'NONE',  ( 22.03867513459498184, 1.110223024625156540E-13, -2.500000000000057732 ) ) ;
#29694=CARTESIAN_POINT ( 'NONE',  ( 14.31250000000002309, -0.8284271247461153509, 2.000000000000151879 ) ) ;
#29697=CARTESIAN_POINT ( 'NONE',  ( 18.47617513459497474, 1.035533905932929599, 2.499999999999844569 ) ) ;
#29726=VECTOR ( 'NONE', #15314, 1000.000000000000000 ) ;
#29752=ORIENTED_EDGE ( 'NONE', *, *, #27785, .T. ) ;
#29753=CARTESIAN_POINT ( 'NONE',  ( 14.12500000000002665, -2.649519052838222866, 0.000000000000000000 ) ) ;
#29780=VERTEX_POINT ( 'NONE', #2831 ) ;
#29807=CARTESIAN_POINT ( 'NONE',  ( 10.00000000000014744, 1.941674212873021999, 0.8547671284023850014 ) ) ;
#29809=VERTEX_POINT ( 'NONE', #29669 ) ;
#29813=ORIENTED_EDGE ( 'NONE', *, *, #29309, .F. ) ;
#29817=CARTESIAN_POINT ( 'NONE',  ( 22.87500000000000711, 1.414213562373312083, -1.414213562373090038 ) ) ;
#29834=CYLINDRICAL_SURFACE ( 'NONE', #14925, 2.499999999999999112 ) ;
#29848=CARTESIAN_POINT ( 'NONE',  ( 11.87500000000007994, 1.414213562373312083, -1.414213562373090038 ) ) ;
#29851=CARTESIAN_POINT ( 'NONE',  ( 10.00000000000014744, 1.820735071450596099, -1.172870270573495910 ) ) ;
#29856=CARTESIAN_POINT ( 'NONE',  ( 24.50844993798688165, 0.4074731033292928184, 2.466641088734008669 ) ) ;
#29859=LINE ( 'NONE', #18525, #10912 ) ;
#29869=CARTESIAN_POINT ( 'NONE',  ( 18.62500000000003197, -1.414213562373034527, -1.414213562373090038 ) ) ;
#29875=ORIENTED_EDGE ( 'NONE', *, *, #10093, .T. ) ;
#29880=VERTEX_POINT ( 'NONE', #10972 ) ;
#29885=ORIENTED_EDGE ( 'NONE', *, *, #809, .F. ) ;
#29890=ORIENTED_EDGE ( 'NONE', *, *, #22818, .T. ) ;
#29905=CARTESIAN_POINT ( 'NONE',  ( 12.00000000000012079, -1.873492889144789952, 1.873492889144845464 ) ) ;
#29921=CARTESIAN_POINT ( 'NONE',  ( 23.18750000000007461, 1.097466725451679892, -2.649519052838358757 ) ) ;
#29922=( BOUNDED_CURVE ( )  B_SPLINE_CURVE ( 2, ( #20707, #2415, #4248, #7168, #4854, #16288, #28046, #2555, #23325 ),
 .UNSPECIFIED., .F., .F. ) 
 B_SPLINE_CURVE_WITH_KNOTS ( ( 3, 2, 2, 2, 3 ),
 ( 0.2031250000000000000, 0.2109375000000000000, 0.2187500000000000000, 0.2265625000000000000, 0.2343750000000000000 ),
 .UNSPECIFIED. ) 
 CURVE ( )  GEOMETRIC_REPRESENTATION_ITEM ( )  RATIONAL_B_SPLINE_CURVE ( ( 1.000000000000000000, 0.9238795325112867385, 1.000000000000000000, 0.9238795325112867385, 1.000000000000000000, 0.9238795325112867385, 1.000000000000000000, 0.9238795325112867385, 1.000000000000000000 ) ) 
 REPRESENTATION_ITEM ( '' )  );
#29928=ORIENTED_EDGE ( 'NONE', *, *, #17345, .T. ) ;
#29929=CARTESIAN_POINT ( 'NONE',  ( 11.37500000000010658, -1.414213562372979016, 1.414213562372979016 ) ) ;
#29944=ORIENTED_EDGE ( 'NONE', *, *, #25590, .F. ) ;
#29945=CARTESIAN_POINT ( 'NONE',  ( 22.50000000000015987, 1.873492889145067508, -1.873492889144956486 ) ) ;
#29968=CARTESIAN_POINT ( 'NONE',  ( 24.56250000000017764, -1.999999999999911626, -0.8284271247462354770 ) ) ;
#29974=CARTESIAN_POINT ( 'NONE',  ( 0.000000000000000000, 0.000000000000000000, 0.000000000000000000 ) ) ;
#29975=FACE_OUTER_BOUND ( 'NONE', #1778, .T. ) ;
#29983=CARTESIAN_POINT ( 'NONE',  ( 16.16367513459493566, 1.767766952966487448, -1.767766952966431937 ) ) ;
#30000=CARTESIAN_POINT ( 'NONE',  ( 11.43750000000003197, -1.999999999999911626, 0.8284271247462955401 ) ) ;
#30001=EDGE_LOOP ( 'NONE', ( #21878, #4198, #14154, #12900 ) ) ;
#30004=CARTESIAN_POINT ( 'NONE',  ( 18.03867513459492145, 1.665334536937734811E-13, -2.500000000000057732 ) ) ;
#30029=CARTESIAN_POINT ( 'NONE',  ( 19.12500000000014211, 1.414213562373256572, 1.414213562373034527 ) ) ;
#30030=LINE ( 'NONE', #18540, #29569 ) ;
#30036=CARTESIAN_POINT ( 'NONE',  ( 11.77382486540525797, 2.500000000000144773, 1.035533905932689347 ) ) ;
#30048=ORIENTED_EDGE ( 'NONE', *, *, #20923, .F. ) ;
#30049=CARTESIAN_POINT ( 'NONE',  ( 13.03867513459488947, 5.551115123125782702E-14, -2.500000000000002220 ) ) ;
#30058=STYLED_ITEM ( 'NONE', ( #15149 ), #1155 ) ;
#30062=CARTESIAN_POINT ( 'NONE',  ( 12.93750000000013145, -1.097466725451499370, 2.649519052838118061 ) ) ;
#30064=CARTESIAN_POINT ( 'NONE',  ( 12.46132486540529882, 1.110223024625156540E-13, -2.500000000000057732 ) ) ;
#30079=CARTESIAN_POINT ( 'NONE',  ( 22.12500000000006040, 1.665334536937734811E-13, -2.649519052838500421 ) ) ;
#30088=CARTESIAN_POINT ( 'NONE',  ( 13.75000000000006750, 2.220446049250313081E-13, -2.000000000000001776 ) ) ;
#30105=CARTESIAN_POINT ( 'NONE',  ( 20.56250000000005684, 2.649519052838298805, -1.097466725451559322 ) ) ;
#30110=DIRECTION ( 'NONE',  ( -1.000000000000000000, -1.665334536937731113E-16, 1.526556658859586792E-16 ) ) ;
#30115=CARTESIAN_POINT ( 'NONE',  ( 10.00000000000017053, -0.2656921846150581690, 2.453244723652735271 ) ) ;
#30125=CARTESIAN_POINT ( 'NONE',  ( 21.18750000000019540, 0.8284271247462955401, 2.000000000000031530 ) ) ;
#30127=EDGE_CURVE ( 'NONE', #29780, #5395, #25584, .T. ) ;
#30134=CARTESIAN_POINT ( 'NONE',  ( 24.70360430863998502, -2.251580690448135247, -0.4762138706651334319 ) ) ;
#30158=CARTESIAN_POINT ( 'NONE',  ( 12.75000000000017764, 1.665334536937734811E-13, -2.000000000000001776 ) ) ;
#30192=CARTESIAN_POINT ( 'NONE',  ( 11.52382486540523132, 1.035533905932869425, -2.500000000000024425 ) ) ;
#30217=CARTESIAN_POINT ( 'NONE',  ( 10.68750000000010658, 2.649519052838419153, 1.097466725451619718 ) ) ;
#30228=EDGE_CURVE ( 'NONE', #24536, #22842, #6555, .T. ) ;
#30233=CARTESIAN_POINT ( 'NONE',  ( 24.06250000000015632, -1.097466725451439196, -2.649519052838419153 ) ) ;
#30252=DIRECTION ( 'NONE',  ( -1.000000000000000000, -1.665334536937731113E-16, 1.526556658859586792E-16 ) ) ;
#30255=CARTESIAN_POINT ( 'NONE',  ( 22.43750000000002842, 1.097466725451559322, -2.649519052838298805 ) ) ;
#30264=CARTESIAN_POINT ( 'NONE',  ( 22.14882486540523132, -2.499999999999964473, 1.035533905932749299 ) ) ;
#30267=( GEOMETRIC_REPRESENTATION_CONTEXT ( 3 ) GLOBAL_UNCERTAINTY_ASSIGNED_CONTEXT ( ( #10708 ) ) GLOBAL_UNIT_ASSIGNED_CONTEXT ( ( #20839, #13963, #25416 ) ) REPRESENTATION_CONTEXT ( 'NONE', 'WORKASPACE' ) );
#30274=B_SPLINE_CURVE_WITH_KNOTS ( 'NONE', 3,
 ( #20787, #22476, #8322, #13138, #10823, #28418, #9407, #2484, #26127, #16507, #18640, #25833, #2344, #27813, #4482, #13906, #12201, #30134, #16656, #16207, #4626, #25678, #23544, #11904, #21237, #14059, #16806, #7248, #23248, #4783 ),
 .UNSPECIFIED., .F., .F.,
 ( 4, 2, 2, 2, 2, 2, 2, 2, 2, 2, 2, 2, 2, 2, 4 ),
 ( 0.0006116782145977108518, 0.001065641339918334783, 0.001519604465238958823, 0.001973567590559582429, 0.002427530715880206469, 0.003335456966521454115, 0.003789420091842078155, 0.004243383217162701761, 0.004697346342483326234, 0.005151309467803949840, 0.006059235718445197920, 0.006513198843765822393, 0.006967161969086445999, 0.007421125094407070473, 0.007875088219727693212 ),
 .UNSPECIFIED. ) ;
#30276=CARTESIAN_POINT ( 'NONE',  ( 10.81250000000010125, -2.649519052838178457, 1.097466725451499370 ) ) ;
#30279=CARTESIAN_POINT ( 'NONE',  ( 24.75000000000010658, 1.665334536937734811E-13, -2.000000000000001776 ) ) ;
#30288=CARTESIAN_POINT ( 'NONE',  ( 16.60117513459497118, -1.035533905932689347, 2.499999999999904521 ) ) ;
#30291=CARTESIAN_POINT ( 'NONE',  ( 15.96132486540519047, 1.665334536937734811E-13, 2.500000000000057732 ) ) ;
#30304=CARTESIAN_POINT ( 'NONE',  ( 20.03867513459486815, 1.665334536937734811E-13, -2.500000000000057732 ) ) ;
#30307=ADVANCED_FACE ( 'NONE', ( #12902 ), #26663, .T. ) ;
#30308=CARTESIAN_POINT ( 'NONE',  ( 21.53867513459484329, 0.000000000000000000, 2.500000000000002220 ) ) ;
#30312=CARTESIAN_POINT ( 'NONE',  ( 14.43750000000014033, -1.999999999999851674, 0.8284271247462955401 ) ) ;
#30337=CARTESIAN_POINT ( 'NONE',  ( 20.31250000000012079, -0.8284271247461152399, 2.000000000000031530 ) ) ;
#30344=CARTESIAN_POINT ( 'NONE',  ( 14.83632486540520290, 1.767766952966376426, 1.767766952966376426 ) ) ;
#30359=CARTESIAN_POINT ( 'NONE',  ( 23.47617513459499250, 1.035533905932809473, 2.499999999999904521 ) ) ;
#30369=VERTEX_POINT ( 'NONE', #30049 ) ;
#30370=CARTESIAN_POINT ( 'NONE',  ( 11.18750000000003908, -2.649519052838238409, -1.097466725451559322 ) ) ;
#30386=CARTESIAN_POINT ( 'NONE',  ( 23.24999999999999289, 1.873492889144956486, -1.873492889144900975 ) ) ;
#30407=CARTESIAN_POINT ( 'NONE',  ( 21.31250000000010658, -1.097466725451379244, -2.649519052838358757 ) ) ;
#30410=FACE_OUTER_BOUND ( 'NONE', #10924, .T. ) ;
ENDSEC;
END-ISO-10303-21;
